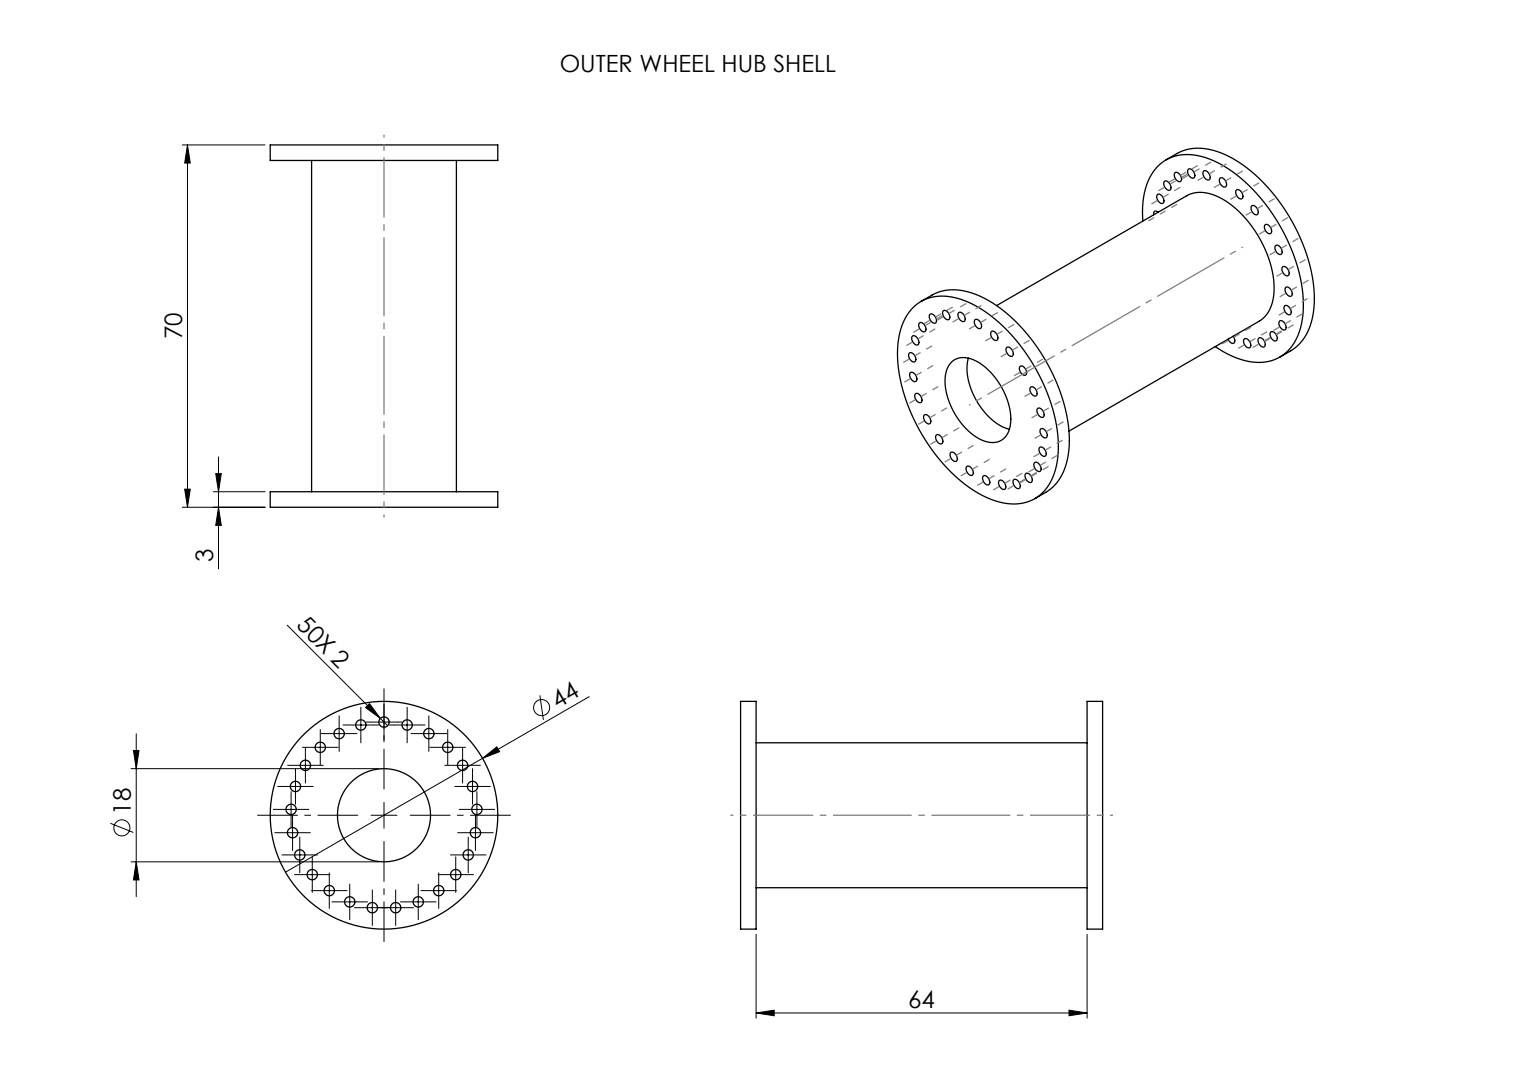
ISO-10303-21;
HEADER;
FILE_DESCRIPTION (('STEP AP214'),
    '1' );
FILE_NAME ('Outer Wheel Hub Shell.step',
    '2026-10-08T05:56:58',
    ( '' ),
    ( '' ),
    'SwSTEP 2.0',
    'SolidWorks 2026',
    '' );
FILE_SCHEMA (( 'AUTOMOTIVE_DESIGN' ));
ENDSEC;

DATA;
#6=ORIENTED_EDGE ( 'NONE', *, *, #9270, .F. ) ;
#16=VECTOR ( 'NONE', #6986, 1000.000000000000000 ) ;
#21=CARTESIAN_POINT ( 'NONE',  ( -14.19790265903626647, 9.644882309621941374, 35.00000000000000000 ) ) ;
#22=VERTEX_POINT ( 'NONE', #14244 ) ;
#27=DIRECTION ( 'NONE',  ( 0.000000000000000000, 0.000000000000000000, 1.000000000000000000 ) ) ;
#28=CARTESIAN_POINT ( 'NONE',  ( -10.58013454126452224, -14.56230589874905235, 32.00000000000000000 ) ) ;
#30=ORIENTED_EDGE ( 'NONE', *, *, #18526, .T. ) ;
#35=ADVANCED_FACE ( 'NONE', ( #2227 ), #2033, .F. ) ;
#38=CARTESIAN_POINT ( 'NONE',  ( 15.28688694438835505, -7.664027248171309203, -32.00000000000000000 ) ) ;
#40=ORIENTED_EDGE ( 'NONE', *, *, #11273, .T. ) ;
#42=ADVANCED_FACE ( 'NONE', ( #15944 ), #11240, .F. ) ;
#44=ORIENTED_EDGE ( 'NONE', *, *, #4692, .F. ) ;
#45=DIRECTION ( 'NONE',  ( 0.000000000000000000, 0.000000000000000000, -1.000000000000000000 ) ) ;
#52=CIRCLE ( 'NONE', #15065, 1.000000000000004441 ) ;
#61=AXIS2_PLACEMENT_3D ( 'NONE', #11825, #841, #14548 ) ;
#65=AXIS2_PLACEMENT_3D ( 'NONE', #16794, #19682, #3071 ) ;
#66=DIRECTION ( 'NONE',  ( -1.000000000000000000, 0.000000000000000000, 0.000000000000000000 ) ) ;
#68=DIRECTION ( 'NONE',  ( 1.000000000000000000, 0.000000000000000000, 0.000000000000000000 ) ) ;
#74=EDGE_CURVE ( 'NONE', #13547, #344, #8025, .T. ) ;
#78=FACE_BOUND ( 'NONE', #16173, .T. ) ;
#84=EDGE_CURVE ( 'NONE', #8438, #18497, #5035, .T. ) ;
#92=AXIS2_PLACEMENT_3D ( 'NONE', #12278, #16979, #66 ) ;
#99=CYLINDRICAL_SURFACE ( 'NONE', #7805, 22.00000000000000355 ) ;
#102=ORIENTED_EDGE ( 'NONE', *, *, #9565, .F. ) ;
#108=CARTESIAN_POINT ( 'NONE',  ( 0.000000000000000000, 0.000000000000000000, 35.00000000000000000 ) ) ;
#110=CARTESIAN_POINT ( 'NONE',  ( 17.11901729331276556, 5.562305898749055011, -32.00000000000000000 ) ) ;
#111=EDGE_CURVE ( 'NONE', #18625, #19430, #2327, .T. ) ;
#124=EDGE_CURVE ( 'NONE', #6609, #1230, #1374, .T. ) ;
#127=EDGE_CURVE ( 'NONE', #15888, #11336, #18737, .T. ) ;
#128=DIRECTION ( 'NONE',  ( 0.000000000000000000, 0.000000000000000000, 1.000000000000000000 ) ) ;
#129=ORIENTED_EDGE ( 'NONE', *, *, #9030, .F. ) ;
#130=DIRECTION ( 'NONE',  ( 1.000000000000000000, 0.000000000000000000, 0.000000000000000000 ) ) ;
#133=DIRECTION ( 'NONE',  ( 1.000000000000000000, 0.000000000000000000, 0.000000000000000000 ) ) ;
#143=DIRECTION ( 'NONE',  ( -0.000000000000000000, -0.000000000000000000, 1.000000000000000000 ) ) ;
#151=ORIENTED_EDGE ( 'NONE', *, *, #9100, .T. ) ;
#152=SHAPE_DEFINITION_REPRESENTATION ( #11949, #13463 ) ;
#155=VERTEX_POINT ( 'NONE', #3633 ) ;
#160=AXIS2_PLACEMENT_3D ( 'NONE', #12502, #14297, #392 ) ;
#165=VECTOR ( 'NONE', #11258, 1000.000000000000000 ) ;
#177=EDGE_LOOP ( 'NONE', ( #14869, #8807, #10159, #6951 ) ) ;
#183=DIRECTION ( 'NONE',  ( 0.000000000000000000, 0.000000000000000000, 1.000000000000000000 ) ) ;
#188=ORIENTED_EDGE ( 'NONE', *, *, #15203, .F. ) ;
#195=CARTESIAN_POINT ( 'NONE',  ( 12.86923836996420967, -11.47363181547641453, 32.00000000000000000 ) ) ;
#205=DIRECTION ( 'NONE',  ( 1.000000000000000000, 0.000000000000000000, 0.000000000000000000 ) ) ;
#209=ADVANCED_FACE ( 'NONE', ( #15358 ), #16764, .F. ) ;
#218=ORIENTED_EDGE ( 'NONE', *, *, #8182, .T. ) ;
#219=CIRCLE ( 'NONE', #8203, 1.000000000000000888 ) ;
#226=VERTEX_POINT ( 'NONE', #15455 ) ;
#228=EDGE_LOOP ( 'NONE', ( #8346, #6074 ) ) ;
#236=DIRECTION ( 'NONE',  ( 1.000000000000000000, 0.000000000000000000, 0.000000000000000000 ) ) ;
#245=ORIENTED_EDGE ( 'NONE', *, *, #12939, .T. ) ;
#257=VERTEX_POINT ( 'NONE', #7635 ) ;
#258=DIRECTION ( 'NONE',  ( 0.000000000000000000, 0.000000000000000000, 1.000000000000000000 ) ) ;
#261=ORIENTED_EDGE ( 'NONE', *, *, #7786, .T. ) ;
#264=FACE_BOUND ( 'NONE', #19064, .T. ) ;
#271=VERTEX_POINT ( 'NONE', #7531 ) ;
#273=AXIS2_PLACEMENT_3D ( 'NONE', #16273, #13173, #8869 ) ;
#277=DIRECTION ( 'NONE',  ( 1.000000000000000000, 0.000000000000000000, 0.000000000000000000 ) ) ;
#286=EDGE_CURVE ( 'NONE', #5172, #4659, #9375, .T. ) ;
#288=AXIS2_PLACEMENT_3D ( 'NONE', #4753, #9067, #13763 ) ;
#293=DIRECTION ( 'NONE',  ( 1.000000000000000000, 0.000000000000000000, 0.000000000000000000 ) ) ;
#295=DIRECTION ( 'NONE',  ( -1.000000000000000000, 0.000000000000000000, 0.000000000000000000 ) ) ;
#297=SURFACE_STYLE_FILL_AREA ( #4139 ) ;
#300=CARTESIAN_POINT ( 'NONE',  ( -18.11901729331277267, 5.562305898749051458, 35.00000000000000000 ) ) ;
#304=LINE ( 'NONE', #1515, #19226 ) ;
#305=CIRCLE ( 'NONE', #5078, 0.9999999999999974465 ) ;
#310=CYLINDRICAL_SURFACE ( 'NONE', #17454, 1.000000000000000888 ) ;
#319=CARTESIAN_POINT ( 'NONE',  ( 5.510910596163084625E-16, 18.00000000000000355, 32.00000000000000000 ) ) ;
#321=ORIENTED_EDGE ( 'NONE', *, *, #19741, .T. ) ;
#325=CYLINDRICAL_SURFACE ( 'NONE', #16943, 1.000000000000000888 ) ;
#330=ORIENTED_EDGE ( 'NONE', *, *, #12182, .F. ) ;
#341=CARTESIAN_POINT ( 'NONE',  ( 5.510910596163084625E-16, 18.00000000000000355, -32.00000000000000000 ) ) ;
#342=EDGE_LOOP ( 'NONE', ( #5793, #6421, #6456, #12755 ) ) ;
#344=VERTEX_POINT ( 'NONE', #2135 ) ;
#350=AXIS2_PLACEMENT_3D ( 'NONE', #15262, #4448, #9055 ) ;
#355=ORIENTED_EDGE ( 'NONE', *, *, #12536, .T. ) ;
#357=CARTESIAN_POINT ( 'NONE',  ( 14.00000000000000178, 1.714505518806294835E-15, -32.00000000000000000 ) ) ;
#360=FACE_OUTER_BOUND ( 'NONE', #7817, .T. ) ;
#362=CARTESIAN_POINT ( 'NONE',  ( 18.68117051311639543, -3.372863662543048591, 35.00000000000000000 ) ) ;
#365=ADVANCED_FACE ( 'NONE', ( #12843 ), #6521, .F. ) ;
#372=AXIS2_PLACEMENT_3D ( 'NONE', #16435, #19135, #4224 ) ;
#383=LINE ( 'NONE', #6367, #16649 ) ;
#388=AXIS2_PLACEMENT_3D ( 'NONE', #15598, #18590, #11093 ) ;
#389=AXIS2_PLACEMENT_3D ( 'NONE', #8278, #3775, #11481 ) ;
#390=CARTESIAN_POINT ( 'NONE',  ( -6.626241948324210540, -16.73597674598852336, 32.00000000000000000 ) ) ;
#392=DIRECTION ( 'NONE',  ( 1.000000000000000000, 0.000000000000000000, 0.000000000000000000 ) ) ;
#402=DIRECTION ( 'NONE',  ( 0.000000000000000000, 0.000000000000000000, -1.000000000000000000 ) ) ;
#404=CYLINDRICAL_SURFACE ( 'NONE', #4852, 1.000000000000004441 ) ;
#412=CIRCLE ( 'NONE', #11553, 1.000000000000004441 ) ;
#417=ORIENTED_EDGE ( 'NONE', *, *, #7596, .F. ) ;
#421=FACE_OUTER_BOUND ( 'NONE', #11319, .T. ) ;
#424=CARTESIAN_POINT ( 'NONE',  ( -9.580134541264520465, -14.56230589874905235, -35.00000000000000000 ) ) ;
#425=AXIS2_PLACEMENT_3D ( 'NONE', #7432, #4154, #17966 ) ;
#430=CARTESIAN_POINT ( 'NONE',  ( 17.68117051311639898, -3.372863662543048591, -32.00000000000000000 ) ) ;
#435=ORIENTED_EDGE ( 'NONE', *, *, #17905, .F. ) ;
#440=EDGE_LOOP ( 'NONE', ( #15883, #17623 ) ) ;
#454=ORIENTED_EDGE ( 'NONE', *, *, #8309, .T. ) ;
#459=ORIENTED_EDGE ( 'NONE', *, *, #7878, .F. ) ;
#468=ORIENTED_EDGE ( 'NONE', *, *, #6736, .T. ) ;
#473=DIRECTION ( 'NONE',  ( 0.000000000000000000, 0.000000000000000000, -1.000000000000000000 ) ) ;
#474=ORIENTED_EDGE ( 'NONE', *, *, #11666, .T. ) ;
#477=AXIS2_PLACEMENT_3D ( 'NONE', #18214, #19704, #4602 ) ;
#478=ORIENTED_EDGE ( 'NONE', *, *, #16286, .F. ) ;
#482=VECTOR ( 'NONE', #13106, 1000.000000000000000 ) ;
#490=ADVANCED_FACE ( 'NONE', ( #16238 ), #3832, .F. ) ;
#497=ORIENTED_EDGE ( 'NONE', *, *, #6656, .F. ) ;
#498=CIRCLE ( 'NONE', #11670, 0.9999999999999974465 ) ;
#499=DIRECTION ( 'NONE',  ( 1.000000000000000000, 0.000000000000000000, 0.000000000000000000 ) ) ;
#505=DIRECTION ( 'NONE',  ( 1.000000000000000000, 0.000000000000000000, 0.000000000000000000 ) ) ;
#511=CARTESIAN_POINT ( 'NONE',  ( 0.000000000000000000, 0.000000000000000000, -30.00000000000000355 ) ) ;
#512=ORIENTED_EDGE ( 'NONE', *, *, #15204, .T. ) ;
#518=FACE_OUTER_BOUND ( 'NONE', #1664, .T. ) ;
#521=CARTESIAN_POINT ( 'NONE',  ( -12.86923836996420611, -11.47363181547641275, 35.00000000000000000 ) ) ;
#524=CARTESIAN_POINT ( 'NONE',  ( -17.96448111170888851, 1.130229351527647585, 32.00000000000000000 ) ) ;
#526=DIRECTION ( 'NONE',  ( 0.000000000000000000, 0.000000000000000000, 1.000000000000000000 ) ) ;
#538=CARTESIAN_POINT ( 'NONE',  ( 12.32184790671639618, 13.12143529358541016, 32.00000000000000000 ) ) ;
#556=ORIENTED_EDGE ( 'NONE', *, *, #11604, .T. ) ;
#557=CARTESIAN_POINT ( 'NONE',  ( -12.00000000000000178, 0.000000000000000000, 35.00000000000000000 ) ) ;
#562=VERTEX_POINT ( 'NONE', #12229 ) ;
#563=DIRECTION ( 'NONE',  ( -0.000000000000000000, -0.000000000000000000, 1.000000000000000000 ) ) ;
#567=CIRCLE ( 'NONE', #11727, 14.00000000000000178 ) ;
#574=FACE_BOUND ( 'NONE', #7715, .T. ) ;
#584=DIRECTION ( 'NONE',  ( 0.000000000000000000, 0.000000000000000000, -1.000000000000000000 ) ) ;
#585=VECTOR ( 'NONE', #11111, 1000.000000000000000 ) ;
#586=ORIENTED_EDGE ( 'NONE', *, *, #6888, .T. ) ;
#587=CARTESIAN_POINT ( 'NONE',  ( -8.671566133830875600, 15.77352024078954429, -35.00000000000000000 ) ) ;
#597=CYLINDRICAL_SURFACE ( 'NONE', #3082, 1.000000000000004441 ) ;
#600=VERTEX_POINT ( 'NONE', #1222 ) ;
#601=CYLINDRICAL_SURFACE ( 'NONE', #13048, 1.000000000000000888 ) ;
#612=CARTESIAN_POINT ( 'NONE',  ( -12.32184790671639085, 13.12143529358541549, -32.00000000000000000 ) ) ;
#613=AXIS2_PLACEMENT_3D ( 'NONE', #10764, #563, #14261 ) ;
#620=CARTESIAN_POINT ( 'NONE',  ( -6.626241948324210540, -16.73597674598852336, -32.00000000000000000 ) ) ;
#625=ORIENTED_EDGE ( 'NONE', *, *, #10006, .T. ) ;
#636=FACE_BOUND ( 'NONE', #2747, .T. ) ;
#642=LINE ( 'NONE', #1837, #19205 ) ;
#649=EDGE_LOOP ( 'NONE', ( #15973, #2519, #13118, #2689 ) ) ;
#656=EDGE_LOOP ( 'NONE', ( #12086, #15329 ) ) ;
#662=EDGE_CURVE ( 'NONE', #16700, #600, #4069, .T. ) ;
#666=ORIENTED_EDGE ( 'NONE', *, *, #14685, .T. ) ;
#669=ADVANCED_FACE ( 'NONE', ( #3317 ), #12722, .F. ) ;
#672=ORIENTED_EDGE ( 'NONE', *, *, #13623, .F. ) ;
#674=LINE ( 'NONE', #2526, #7891 ) ;
#676=VERTEX_POINT ( 'NONE', #5011 ) ;
#705=ORIENTED_EDGE ( 'NONE', *, *, #2287, .T. ) ;
#711=ORIENTED_EDGE ( 'NONE', *, *, #7911, .F. ) ;
#716=AXIS2_PLACEMENT_3D ( 'NONE', #3976, #1170, #14686 ) ;
#718=CARTESIAN_POINT ( 'NONE',  ( 9.671566133830877376, 15.77352024078954784, -32.00000000000000000 ) ) ;
#722=FILL_AREA_STYLE_COLOUR ( '', #9371 ) ;
#726=DIRECTION ( 'NONE',  ( -1.000000000000000000, 0.000000000000000000, 0.000000000000000000 ) ) ;
#733=DIRECTION ( 'NONE',  ( 0.000000000000000000, 0.000000000000000000, -1.000000000000000000 ) ) ;
#735=DIRECTION ( 'NONE',  ( 1.000000000000000000, 0.000000000000000000, 0.000000000000000000 ) ) ;
#738=FACE_BOUND ( 'NONE', #4707, .T. ) ;
#742=CARTESIAN_POINT ( 'NONE',  ( -11.58013454126452579, -14.56230589874905235, -32.00000000000000000 ) ) ;
#743=DIRECTION ( 'NONE',  ( 0.000000000000000000, 0.000000000000000000, -1.000000000000000000 ) ) ;
#744=EDGE_CURVE ( 'NONE', #18193, #12621, #16104, .T. ) ;
#749=DIRECTION ( 'NONE',  ( 1.000000000000000000, 0.000000000000000000, 0.000000000000000000 ) ) ;
#753=AXIS2_PLACEMENT_3D ( 'NONE', #9858, #9653, #15648 ) ;
#764=ORIENTED_EDGE ( 'NONE', *, *, #5632, .T. ) ;
#770=CARTESIAN_POINT ( 'NONE',  ( -18.96448111170889206, 1.130229351527647585, -35.00000000000000000 ) ) ;
#771=DIRECTION ( 'NONE',  ( 0.000000000000000000, 0.000000000000000000, 1.000000000000000000 ) ) ;
#792=DIRECTION ( 'NONE',  ( 0.000000000000000000, 0.000000000000000000, 1.000000000000000000 ) ) ;
#797=CARTESIAN_POINT ( 'NONE',  ( -15.19790265903627180, 9.644882309621941374, 35.00000000000000000 ) ) ;
#799=CARTESIAN_POINT ( 'NONE',  ( -9.000000000000001776, 0.000000000000000000, -30.00000000000000355 ) ) ;
#823=DIRECTION ( 'NONE',  ( 1.000000000000000000, 0.000000000000000000, 0.000000000000000000 ) ) ;
#829=CARTESIAN_POINT ( 'NONE',  ( -16.28688694438836038, -7.664027248171298545, -32.00000000000000000 ) ) ;
#833=DIRECTION ( 'NONE',  ( -0.000000000000000000, -0.000000000000000000, 1.000000000000000000 ) ) ;
#834=AXIS2_PLACEMENT_3D ( 'NONE', #19075, #17680, #9988 ) ;
#837=FACE_BOUND ( 'NONE', #6605, .T. ) ;
#841=DIRECTION ( 'NONE',  ( -0.000000000000000000, -0.000000000000000000, 1.000000000000000000 ) ) ;
#846=FACE_BOUND ( 'NONE', #14940, .T. ) ;
#855=DIRECTION ( 'NONE',  ( 1.000000000000000000, 0.000000000000000000, 0.000000000000000000 ) ) ;
#857=ORIENTED_EDGE ( 'NONE', *, *, #17755, .F. ) ;
#865=DIRECTION ( 'NONE',  ( 0.000000000000000000, 0.000000000000000000, -1.000000000000000000 ) ) ;
#888=CARTESIAN_POINT ( 'NONE',  ( 3.476417968967386418, 17.43449690031536292, 32.00000000000000000 ) ) ;
#894=AXIS2_PLACEMENT_3D ( 'NONE', #13584, #13287, #16392 ) ;
#907=AXIS2_PLACEMENT_3D ( 'NONE', #1856, #14055, #13963 ) ;
#912=DIRECTION ( 'NONE',  ( 1.000000000000000000, 0.000000000000000000, 0.000000000000000000 ) ) ;
#916=ORIENTED_EDGE ( 'NONE', *, *, #8748, .F. ) ;
#928=DIRECTION ( 'NONE',  ( -1.000000000000000000, 0.000000000000000000, 0.000000000000000000 ) ) ;
#929=ORIENTED_EDGE ( 'NONE', *, *, #16286, .T. ) ;
#932=DIRECTION ( 'NONE',  ( 1.000000000000000000, 0.000000000000000000, 0.000000000000000000 ) ) ;
#933=AXIS2_PLACEMENT_3D ( 'NONE', #6535, #2148, #5051 ) ;
#936=DIRECTION ( 'NONE',  ( 1.000000000000000000, 0.000000000000000000, 0.000000000000000000 ) ) ;
#937=CARTESIAN_POINT ( 'NONE',  ( 0.000000000000000000, 0.000000000000000000, 35.00000000000000000 ) ) ;
#943=DIRECTION ( 'NONE',  ( 0.000000000000000000, 0.000000000000000000, -1.000000000000000000 ) ) ;
#945=LINE ( 'NONE', #13146, #9312 ) ;
#949=DIRECTION ( 'NONE',  ( -0.000000000000000000, -0.000000000000000000, 1.000000000000000000 ) ) ;
#953=ORIENTED_EDGE ( 'NONE', *, *, #8960, .T. ) ;
#961=ORIENTED_EDGE ( 'NONE', *, *, #11015, .T. ) ;
#962=CARTESIAN_POINT ( 'NONE',  ( 18.68117051311639543, -3.372863662543048591, 32.00000000000000000 ) ) ;
#963=CIRCLE ( 'NONE', #1919, 1.000000000000000888 ) ;
#967=DIRECTION ( 'NONE',  ( -1.000000000000000000, 0.000000000000000000, 0.000000000000000000 ) ) ;
#968=ORIENTED_EDGE ( 'NONE', *, *, #18592, .F. ) ;
#970=LINE ( 'NONE', #17684, #14905 ) ;
#971=ORIENTED_EDGE ( 'NONE', *, *, #4682, .F. ) ;
#982=DIRECTION ( 'NONE',  ( 0.000000000000000000, 0.000000000000000000, 1.000000000000000000 ) ) ;
#983=ORIENTED_EDGE ( 'NONE', *, *, #2761, .F. ) ;
#984=DIRECTION ( 'NONE',  ( 1.000000000000000000, 0.000000000000000000, 0.000000000000000000 ) ) ;
#996=ORIENTED_EDGE ( 'NONE', *, *, #13001, .F. ) ;
#1006=ORIENTED_EDGE ( 'NONE', *, *, #16529, .F. ) ;
#1009=CARTESIAN_POINT ( 'NONE',  ( 1.255998204157470211, -17.85806462366060288, 32.00000000000000000 ) ) ;
#1014=FACE_BOUND ( 'NONE', #7800, .T. ) ;
#1017=ORIENTED_EDGE ( 'NONE', *, *, #19676, .T. ) ;
#1019=EDGE_CURVE ( 'NONE', #15780, #17520, #11302, .T. ) ;
#1024=ORIENTED_EDGE ( 'NONE', *, *, #3666, .F. ) ;
#1027=ADVANCED_FACE ( 'NONE', ( #17294 ), #1697, .F. ) ;
#1028=FACE_OUTER_BOUND ( 'NONE', #19195, .T. ) ;
#1036=VECTOR ( 'NONE', #16677, 1000.000000000000000 ) ;
#1041=VERTEX_POINT ( 'NONE', #3291 ) ;
#1042=DIRECTION ( 'NONE',  ( -0.000000000000000000, -0.000000000000000000, 1.000000000000000000 ) ) ;
#1045=EDGE_LOOP ( 'NONE', ( #18049, #2720, #5129, #19018 ) ) ;
#1058=EDGE_LOOP ( 'NONE', ( #17820, #7756, #19150, #14489 ) ) ;
#1064=DIRECTION ( 'NONE',  ( 0.000000000000000000, 0.000000000000000000, 1.000000000000000000 ) ) ;
#1065=MECHANICAL_DESIGN_GEOMETRIC_PRESENTATION_REPRESENTATION('',(#9705),#3287);
#1066=EDGE_CURVE ( 'NONE', #1381, #19705, #15773, .T. ) ;
#1071=DIRECTION ( 'NONE',  ( 0.000000000000000000, 0.000000000000000000, -1.000000000000000000 ) ) ;
#1074=CARTESIAN_POINT ( 'NONE',  ( 15.19790265903627358, 9.644882309621939598, 32.00000000000000000 ) ) ;
#1076=CARTESIAN_POINT ( 'NONE',  ( -14.86923836996421144, -11.47363181547641275, 35.00000000000000000 ) ) ;
#1079=CARTESIAN_POINT ( 'NONE',  ( -13.86923836996420967, -11.47363181547641275, 32.00000000000000000 ) ) ;
#1084=CARTESIAN_POINT ( 'NONE',  ( 17.68117051311639898, -3.372863662543048591, 35.00000000000000000 ) ) ;
#1095=ORIENTED_EDGE ( 'NONE', *, *, #14831, .F. ) ;
#1098=DIRECTION ( 'NONE',  ( 1.000000000000000000, 0.000000000000000000, 0.000000000000000000 ) ) ;
#1101=CIRCLE ( 'NONE', #14213, 12.00000000000000178 ) ;
#1108=AXIS2_PLACEMENT_3D ( 'NONE', #4038, #19235, #5530 ) ;
#1115=CIRCLE ( 'NONE', #11348, 1.000000000000004441 ) ;
#1116=CARTESIAN_POINT ( 'NONE',  ( 17.96448111170888851, 1.130229351527639148, 35.00000000000000000 ) ) ;
#1117=DIRECTION ( 'NONE',  ( -1.000000000000000000, 0.000000000000000000, 0.000000000000000000 ) ) ;
#1124=ORIENTED_EDGE ( 'NONE', *, *, #12744, .T. ) ;
#1125=EDGE_CURVE ( 'NONE', #3988, #14268, #7776, .T. ) ;
#1129=VERTEX_POINT ( 'NONE', #6182 ) ;
#1143=EDGE_CURVE ( 'NONE', #7513, #15780, #9300, .T. ) ;
#1149=EDGE_CURVE ( 'NONE', #19757, #19457, #12600, .T. ) ;
#1151=DIRECTION ( 'NONE',  ( 1.000000000000000000, 0.000000000000000000, 0.000000000000000000 ) ) ;
#1152=AXIS2_PLACEMENT_3D ( 'NONE', #13149, #10064, #16167 ) ;
#1154=CARTESIAN_POINT ( 'NONE',  ( 17.11901729331276556, 5.562305898749055011, -35.00000000000000000 ) ) ;
#1161=ORIENTED_EDGE ( 'NONE', *, *, #6150, .T. ) ;
#1163=DIRECTION ( 'NONE',  ( 1.000000000000000000, 0.000000000000000000, 0.000000000000000000 ) ) ;
#1167=ORIENTED_EDGE ( 'NONE', *, *, #17905, .T. ) ;
#1170=DIRECTION ( 'NONE',  ( -0.000000000000000000, -0.000000000000000000, 1.000000000000000000 ) ) ;
#1172=ORIENTED_EDGE ( 'NONE', *, *, #662, .F. ) ;
#1175=CIRCLE ( 'NONE', #9821, 1.000000000000004441 ) ;
#1176=DIRECTION ( 'NONE',  ( 0.000000000000000000, 0.000000000000000000, -1.000000000000000000 ) ) ;
#1182=ORIENTED_EDGE ( 'NONE', *, *, #6055, .F. ) ;
#1183=FACE_OUTER_BOUND ( 'NONE', #8230, .T. ) ;
#1192=AXIS2_PLACEMENT_3D ( 'NONE', #12017, #18122, #12117 ) ;
#1194=DIRECTION ( 'NONE',  ( 1.000000000000000000, 0.000000000000000000, 0.000000000000000000 ) ) ;
#1202=DIRECTION ( 'NONE',  ( 1.000000000000000000, 0.000000000000000000, 0.000000000000000000 ) ) ;
#1203=CARTESIAN_POINT ( 'NONE',  ( -9.580134541264520465, -14.56230589874905235, -32.00000000000000000 ) ) ;
#1207=VERTEX_POINT ( 'NONE', #9905 ) ;
#1213=CYLINDRICAL_SURFACE ( 'NONE', #12720, 0.9999999999999974465 ) ;
#1216=DIRECTION ( 'NONE',  ( 1.000000000000000000, 0.000000000000000000, 0.000000000000000000 ) ) ;
#1220=CIRCLE ( 'NONE', #15590, 1.000000000000000000 ) ;
#1222=CARTESIAN_POINT ( 'NONE',  ( 1.000000000000003331, 18.00000000000000355, -32.00000000000000000 ) ) ;
#1225=CARTESIAN_POINT ( 'NONE',  ( -5.476417968967388639, 17.43449690031536292, 35.00000000000000000 ) ) ;
#1230=VERTEX_POINT ( 'NONE', #16099 ) ;
#1245=ORIENTED_EDGE ( 'NONE', *, *, #9812, .F. ) ;
#1249=CARTESIAN_POINT ( 'NONE',  ( -16.11901729331276911, 5.562305898749051458, -32.00000000000000000 ) ) ;
#1254=ORIENTED_EDGE ( 'NONE', *, *, #6270, .F. ) ;
#1260=EDGE_LOOP ( 'NONE', ( #13516, #17218, #40, #9749 ) ) ;
#1261=CYLINDRICAL_SURFACE ( 'NONE', #273, 1.000000000000004441 ) ;
#1268=DIRECTION ( 'NONE',  ( 1.000000000000000000, 0.000000000000000000, 0.000000000000000000 ) ) ;
#1273=CARTESIAN_POINT ( 'NONE',  ( 17.96448111170888851, 1.130229351527639148, 32.00000000000000000 ) ) ;
#1276=ADVANCED_FACE ( 'NONE', ( #9805 ), #15898, .F. ) ;
#1280=AXIS2_PLACEMENT_3D ( 'NONE', #15135, #2719, #4426 ) ;
#1285=FACE_BOUND ( 'NONE', #3109, .T. ) ;
#1286=DIRECTION ( 'NONE',  ( -0.000000000000000000, -0.000000000000000000, 1.000000000000000000 ) ) ;
#1289=ORIENTED_EDGE ( 'NONE', *, *, #15396, .F. ) ;
#1290=DIRECTION ( 'NONE',  ( 1.000000000000000000, 0.000000000000000000, 0.000000000000000000 ) ) ;
#1294=MECHANICAL_DESIGN_GEOMETRIC_PRESENTATION_REPRESENTATION('',(#18875),#16321);
#1307=VECTOR ( 'NONE', #11955, 1000.000000000000000 ) ;
#1310=DIRECTION ( 'NONE',  ( 1.000000000000000000, 0.000000000000000000, 0.000000000000000000 ) ) ;
#1326=ORIENTED_EDGE ( 'NONE', *, *, #18116, .T. ) ;
#1329=CARTESIAN_POINT ( 'NONE',  ( 9.580134541264516912, -14.56230589874905412, 32.00000000000000000 ) ) ;
#1332=DIRECTION ( 'NONE',  ( 1.000000000000000000, 0.000000000000000000, 0.000000000000000000 ) ) ;
#1348=DIRECTION ( 'NONE',  ( 1.000000000000000000, 0.000000000000000000, 0.000000000000000000 ) ) ;
#1355=DIRECTION ( 'NONE',  ( 0.000000000000000000, 0.000000000000000000, 1.000000000000000000 ) ) ;
#1356=ORIENTED_EDGE ( 'NONE', *, *, #6888, .F. ) ;
#1374=CIRCLE ( 'NONE', #3610, 1.000000000000000888 ) ;
#1381=VERTEX_POINT ( 'NONE', #7657 ) ;
#1383=CARTESIAN_POINT ( 'NONE',  ( 17.11901729331276556, 5.562305898749055011, -32.00000000000000000 ) ) ;
#1386=FACE_BOUND ( 'NONE', #8709, .T. ) ;
#1401=CARTESIAN_POINT ( 'NONE',  ( 17.28688694438834972, -7.664027248171309203, -32.00000000000000000 ) ) ;
#1405=ORIENTED_EDGE ( 'NONE', *, *, #10886, .T. ) ;
#1409=ORIENTED_EDGE ( 'NONE', *, *, #16598, .F. ) ;
#1433=CARTESIAN_POINT ( 'NONE',  ( -17.28688694438836393, -7.664027248171298545, 32.00000000000000000 ) ) ;
#1436=CARTESIAN_POINT ( 'NONE',  ( 16.68117051311640253, -3.372863662543048591, -32.00000000000000000 ) ) ;
#1440=EDGE_LOOP ( 'NONE', ( #2226, #11290, #7945, #5008 ) ) ;
#1441=DIRECTION ( 'NONE',  ( 1.000000000000000000, 0.000000000000000000, 0.000000000000000000 ) ) ;
#1445=EDGE_LOOP ( 'NONE', ( #3057, #18115, #929, #13564 ) ) ;
#1453=CARTESIAN_POINT ( 'NONE',  ( -7.671566133830872047, 15.77352024078954429, -32.00000000000000000 ) ) ;
#1459=DIRECTION ( 'NONE',  ( -0.000000000000000000, -0.000000000000000000, 1.000000000000000000 ) ) ;
#1466=DIRECTION ( 'NONE',  ( 0.000000000000000000, 0.000000000000000000, 1.000000000000000000 ) ) ;
#1470=DIRECTION ( 'NONE',  ( 1.000000000000000000, 0.000000000000000000, 0.000000000000000000 ) ) ;
#1479=FACE_OUTER_BOUND ( 'NONE', #9021, .T. ) ;
#1481=EDGE_CURVE ( 'NONE', #16968, #11811, #3329, .T. ) ;
#1482=CARTESIAN_POINT ( 'NONE',  ( 16.68117051311640253, -3.372863662543048591, -35.00000000000000000 ) ) ;
#1484=CARTESIAN_POINT ( 'NONE',  ( -16.11901729331276911, 5.562305898749051458, -32.00000000000000000 ) ) ;
#1495=VECTOR ( 'NONE', #5397, 1000.000000000000000 ) ;
#1500=EDGE_CURVE ( 'NONE', #17152, #9970, #8733, .T. ) ;
#1506=ORIENTED_EDGE ( 'NONE', *, *, #7570, .F. ) ;
#1509=DIRECTION ( 'NONE',  ( 0.000000000000000000, 0.000000000000000000, 1.000000000000000000 ) ) ;
#1511=DIRECTION ( 'NONE',  ( -1.000000000000000000, 0.000000000000000000, 0.000000000000000000 ) ) ;
#1515=CARTESIAN_POINT ( 'NONE',  ( 13.32184790671640151, 13.12143529358541016, 32.00000000000000000 ) ) ;
#1540=VERTEX_POINT ( 'NONE', #11540 ) ;
#1541=LINE ( 'NONE', #8480, #8395 ) ;
#1543=ORIENTED_EDGE ( 'NONE', *, *, #18666, .T. ) ;
#1544=ADVANCED_FACE ( 'NONE', ( #8450, #2523, #8633, #17836, #13425, #8542, #11832, #10345, #17940, #6924, #14553, #4229, #7304, #19523, #5815, #13045, #846, #16049, #14741, #11636, #2335, #17645, #4035, #3935, #10054, #1028, #16155 ), #14650, .T. ) ;
#1545=CARTESIAN_POINT ( 'NONE',  ( -16.28688694438836038, -7.664027248171298545, -35.00000000000000000 ) ) ;
#1561=VERTEX_POINT ( 'NONE', #4622 ) ;
#1564=ORIENTED_EDGE ( 'NONE', *, *, #9722, .T. ) ;
#1571=CIRCLE ( 'NONE', #15323, 1.000000000000002665 ) ;
#1579=FACE_BOUND ( 'NONE', #13672, .T. ) ;
#1594=EDGE_CURVE ( 'NONE', #15562, #8927, #9328, .T. ) ;
#1598=CARTESIAN_POINT ( 'NONE',  ( 9.000000000000001776, 1.102182119232617911E-15, -35.00000000000000000 ) ) ;
#1604=CARTESIAN_POINT ( 'NONE',  ( -12.32184790671639085, 13.12143529358541549, 35.00000000000000000 ) ) ;
#1622=ORIENTED_EDGE ( 'NONE', *, *, #5804, .T. ) ;
#1629=FACE_OUTER_BOUND ( 'NONE', #12937, .T. ) ;
#1632=EDGE_CURVE ( 'NONE', #7691, #8343, #10533, .T. ) ;
#1642=CARTESIAN_POINT ( 'NONE',  ( 2.255998204157473097, -17.85806462366060288, 32.00000000000000000 ) ) ;
#1643=ORIENTED_EDGE ( 'NONE', *, *, #12286, .T. ) ;
#1650=ORIENTED_EDGE ( 'NONE', *, *, #6270, .T. ) ;
#1651=PRODUCT_CONTEXT ( 'NONE', #13526, 'mechanical' ) ;
#1655=CIRCLE ( 'NONE', #5170, 1.000000000000002442 ) ;
#1657=EDGE_LOOP ( 'NONE', ( #2120, #15431 ) ) ;
#1664=EDGE_LOOP ( 'NONE', ( #2409, #12739, #5086, #102 ) ) ;
#1666=AXIS2_PLACEMENT_3D ( 'NONE', #16616, #18123, #1117 ) ;
#1668=CARTESIAN_POINT ( 'NONE',  ( -5.626241948324210540, -16.73597674598852336, -32.00000000000000000 ) ) ;
#1673=ORIENTED_EDGE ( 'NONE', *, *, #1481, .F. ) ;
#1678=ORIENTED_EDGE ( 'NONE', *, *, #6386, .F. ) ;
#1681=FACE_BOUND ( 'NONE', #14139, .T. ) ;
#1690=CARTESIAN_POINT ( 'NONE',  ( -14.86923836996421144, -11.47363181547641275, -32.00000000000000000 ) ) ;
#1697=CYLINDRICAL_SURFACE ( 'NONE', #17693, 1.000000000000005995 ) ;
#1703=CIRCLE ( 'NONE', #18636, 1.000000000000000888 ) ;
#1704=DIRECTION ( 'NONE',  ( 1.000000000000000000, 0.000000000000000000, 0.000000000000000000 ) ) ;
#1710=EDGE_CURVE ( 'NONE', #7772, #12395, #17396, .T. ) ;
#1720=VECTOR ( 'NONE', #1790, 1000.000000000000000 ) ;
#1724=DIRECTION ( 'NONE',  ( 0.000000000000000000, 0.000000000000000000, 1.000000000000000000 ) ) ;
#1728=EDGE_LOOP ( 'NONE', ( #2809, #13632, #15230, #15114 ) ) ;
#1731=DIRECTION ( 'NONE',  ( -0.000000000000000000, -0.000000000000000000, 1.000000000000000000 ) ) ;
#1732=DIRECTION ( 'NONE',  ( 0.000000000000000000, 0.000000000000000000, 1.000000000000000000 ) ) ;
#1737=ORIENTED_EDGE ( 'NONE', *, *, #18205, .F. ) ;
#1757=ORIENTED_EDGE ( 'NONE', *, *, #3055, .F. ) ;
#1761=ADVANCED_FACE ( 'NONE', ( #4820 ), #10928, .T. ) ;
#1764=DIRECTION ( 'NONE',  ( 1.000000000000000000, 0.000000000000000000, 0.000000000000000000 ) ) ;
#1765=AXIS2_PLACEMENT_3D ( 'NONE', #19492, #4393, #14903 ) ;
#1769=FACE_BOUND ( 'NONE', #11928, .T. ) ;
#1770=EDGE_LOOP ( 'NONE', ( #17052, #10177, #1780, #9726 ) ) ;
#1772=ORIENTED_EDGE ( 'NONE', *, *, #12734, .F. ) ;
#1774=CARTESIAN_POINT ( 'NONE',  ( 3.476417968967386418, 17.43449690031536292, -32.00000000000000000 ) ) ;
#1776=CARTESIAN_POINT ( 'NONE',  ( 12.32184790671639618, 13.12143529358541016, 35.00000000000000000 ) ) ;
#1777=AXIS2_PLACEMENT_3D ( 'NONE', #9171, #18934, #7926 ) ;
#1778=DIRECTION ( 'NONE',  ( 0.000000000000000000, 0.000000000000000000, 1.000000000000000000 ) ) ;
#1780=ORIENTED_EDGE ( 'NONE', *, *, #2004, .F. ) ;
#1783=ORIENTED_EDGE ( 'NONE', *, *, #13211, .F. ) ;
#1787=AXIS2_PLACEMENT_3D ( 'NONE', #3934, #10053, #936 ) ;
#1788=AXIS2_PLACEMENT_3D ( 'NONE', #612, #14017, #9523 ) ;
#1790=DIRECTION ( 'NONE',  ( 0.000000000000000000, 0.000000000000000000, 1.000000000000000000 ) ) ;
#1798=DIRECTION ( 'NONE',  ( 0.000000000000000000, 0.000000000000000000, 1.000000000000000000 ) ) ;
#1804=DIRECTION ( 'NONE',  ( 0.000000000000000000, 0.000000000000000000, 1.000000000000000000 ) ) ;
#1805=CIRCLE ( 'NONE', #9819, 1.000000000000002665 ) ;
#1812=DIRECTION ( 'NONE',  ( 0.000000000000000000, 0.000000000000000000, 1.000000000000000000 ) ) ;
#1813=EDGE_CURVE ( 'NONE', #6546, #2248, #12933, .T. ) ;
#1814=DIRECTION ( 'NONE',  ( -0.000000000000000000, -0.000000000000000000, 1.000000000000000000 ) ) ;
#1825=EDGE_LOOP ( 'NONE', ( #3083, #7794, #8665, #12430 ) ) ;
#1827=EDGE_CURVE ( 'NONE', #15645, #7691, #1101, .T. ) ;
#1832=DIRECTION ( 'NONE',  ( -1.000000000000000000, 0.000000000000000000, 0.000000000000000000 ) ) ;
#1833=AXIS2_PLACEMENT_3D ( 'NONE', #2667, #13476, #5869 ) ;
#1837=CARTESIAN_POINT ( 'NONE',  ( -9.000000000000001776, 0.000000000000000000, -30.00000000000000355 ) ) ;
#1840=EDGE_CURVE ( 'NONE', #11336, #8576, #19311, .T. ) ;
#1843=CARTESIAN_POINT ( 'NONE',  ( -18.11901729331277267, 5.562305898749051458, 32.00000000000000000 ) ) ;
#1845=DIRECTION ( 'NONE',  ( 0.000000000000000000, 0.000000000000000000, 1.000000000000000000 ) ) ;
#1847=CIRCLE ( 'NONE', #12704, 0.9999999999999974465 ) ;
#1848=ORIENTED_EDGE ( 'NONE', *, *, #17371, .F. ) ;
#1851=CIRCLE ( 'NONE', #14319, 1.000000000000004441 ) ;
#1855=EDGE_CURVE ( 'NONE', #10657, #10470, #19632, .T. ) ;
#1856=CARTESIAN_POINT ( 'NONE',  ( -10.58013454126452224, -14.56230589874905235, 35.00000000000000000 ) ) ;
#1861=ORIENTED_EDGE ( 'NONE', *, *, #5100, .F. ) ;
#1862=VECTOR ( 'NONE', #10499, 1000.000000000000000 ) ;
#1866=PLANE ( 'NONE',  #10369 ) ;
#1868=DIRECTION ( 'NONE',  ( 1.000000000000000000, 0.000000000000000000, 0.000000000000000000 ) ) ;
#1885=EDGE_CURVE ( 'NONE', #6940, #19582, #10071, .T. ) ;
#1890=ORIENTED_EDGE ( 'NONE', *, *, #9297, .F. ) ;
#1895=DIRECTION ( 'NONE',  ( 0.000000000000000000, 0.000000000000000000, 1.000000000000000000 ) ) ;
#1900=FACE_OUTER_BOUND ( 'NONE', #14171, .T. ) ;
#1919=AXIS2_PLACEMENT_3D ( 'NONE', #3428, #13935, #130 ) ;
#1920=EDGE_CURVE ( 'NONE', #16239, #12779, #9104, .T. ) ;
#1924=DIRECTION ( 'NONE',  ( 1.000000000000000000, 0.000000000000000000, 0.000000000000000000 ) ) ;
#1930=VECTOR ( 'NONE', #15016, 1000.000000000000000 ) ;
#1931=CARTESIAN_POINT ( 'NONE',  ( 17.96448111170888851, 1.130229351527639148, -32.00000000000000000 ) ) ;
#1932=ADVANCED_FACE ( 'NONE', ( #18310 ), #5989, .F. ) ;
#1935=ORIENTED_EDGE ( 'NONE', *, *, #10207, .F. ) ;
#1936=FACE_OUTER_BOUND ( 'NONE', #18621, .T. ) ;
#1939=CARTESIAN_POINT ( 'NONE',  ( -9.000000000000000000, 1.102182119232617714E-15, 29.00000000000000355 ) ) ;
#1950=ORIENTED_EDGE ( 'NONE', *, *, #11138, .T. ) ;
#1952=ADVANCED_FACE ( 'NONE', ( #10804 ), #99, .T. ) ;
#1955=EDGE_CURVE ( 'NONE', #6290, #5305, #9110, .T. ) ;
#1956=EDGE_CURVE ( 'NONE', #12131, #9602, #15813, .T. ) ;
#1958=AXIS2_PLACEMENT_3D ( 'NONE', #3030, #7628, #1441 ) ;
#1961=DIRECTION ( 'NONE',  ( -1.000000000000000000, 0.000000000000000000, 0.000000000000000000 ) ) ;
#1962=FACE_BOUND ( 'NONE', #8956, .T. ) ;
#1966=EDGE_LOOP ( 'NONE', ( #4725, #9031 ) ) ;
#1976=CARTESIAN_POINT ( 'NONE',  ( 0.000000000000000000, 0.000000000000000000, -30.00000000000000355 ) ) ;
#1977=VERTEX_POINT ( 'NONE', #1598 ) ;
#1979=ADVANCED_FACE ( 'NONE', ( #10512 ), #15111, .F. ) ;
#1983=DIRECTION ( 'NONE',  ( 1.000000000000000000, 0.000000000000000000, 0.000000000000000000 ) ) ;
#1987=CIRCLE ( 'NONE', #12226, 0.9999999999999974465 ) ;
#1990=CIRCLE ( 'NONE', #3591, 1.000000000000004441 ) ;
#1999=DIRECTION ( 'NONE',  ( 1.000000000000000000, 0.000000000000000000, 0.000000000000000000 ) ) ;
#2004=EDGE_CURVE ( 'NONE', #10647, #18235, #14855, .T. ) ;
#2012=DIRECTION ( 'NONE',  ( 1.000000000000000000, 0.000000000000000000, 0.000000000000000000 ) ) ;
#2023=VERTEX_POINT ( 'NONE', #1203 ) ;
#2024=DIRECTION ( 'NONE',  ( 0.000000000000000000, 0.000000000000000000, 1.000000000000000000 ) ) ;
#2025=DIRECTION ( 'NONE',  ( 0.000000000000000000, 0.000000000000000000, -1.000000000000000000 ) ) ;
#2033=CYLINDRICAL_SURFACE ( 'NONE', #12562, 1.000000000000000888 ) ;
#2034=DIRECTION ( 'NONE',  ( -0.000000000000000000, -0.000000000000000000, 1.000000000000000000 ) ) ;
#2036=ORIENTED_EDGE ( 'NONE', *, *, #17824, .T. ) ;
#2047=ORIENTED_EDGE ( 'NONE', *, *, #2731, .F. ) ;
#2064=VECTOR ( 'NONE', #19500, 1000.000000000000000 ) ;
#2073=ORIENTED_EDGE ( 'NONE', *, *, #10828, .T. ) ;
#2087=DIRECTION ( 'NONE',  ( 1.000000000000000000, 0.000000000000000000, 0.000000000000000000 ) ) ;
#2088=CIRCLE ( 'NONE', #4975, 1.000000000000002442 ) ;
#2091=ADVANCED_FACE ( 'NONE', ( #17202 ), #11099, .F. ) ;
#2092=DIRECTION ( 'NONE',  ( 0.000000000000000000, 0.000000000000000000, 1.000000000000000000 ) ) ;
#2097=EDGE_CURVE ( 'NONE', #4232, #5897, #15500, .T. ) ;
#2098=DIRECTION ( 'NONE',  ( 0.000000000000000000, 0.000000000000000000, -1.000000000000000000 ) ) ;
#2100=ORIENTED_EDGE ( 'NONE', *, *, #7221, .T. ) ;
#2103=CIRCLE ( 'NONE', #8817, 1.000000000000003553 ) ;
#2104=ORIENTED_EDGE ( 'NONE', *, *, #10242, .T. ) ;
#2106=CIRCLE ( 'NONE', #1777, 1.000000000000004441 ) ;
#2107=EDGE_CURVE ( 'NONE', #13012, #3997, #1115, .T. ) ;
#2113=ADVANCED_FACE ( 'NONE', ( #4992 ), #15699, .F. ) ;
#2116=DIRECTION ( 'NONE',  ( 0.000000000000000000, 0.000000000000000000, -1.000000000000000000 ) ) ;
#2120=ORIENTED_EDGE ( 'NONE', *, *, #16487, .T. ) ;
#2123=LINE ( 'NONE', #9640, #15256 ) ;
#2127=FACE_BOUND ( 'NONE', #19598, .T. ) ;
#2129=ORIENTED_EDGE ( 'NONE', *, *, #10476, .T. ) ;
#2131=AXIS2_PLACEMENT_3D ( 'NONE', #17009, #14003, #293 ) ;
#2135=CARTESIAN_POINT ( 'NONE',  ( -11.58013454126452579, -14.56230589874905235, -35.00000000000000000 ) ) ;
#2145=ORIENTED_EDGE ( 'NONE', *, *, #5100, .T. ) ;
#2148=DIRECTION ( 'NONE',  ( -0.000000000000000000, -0.000000000000000000, 1.000000000000000000 ) ) ;
#2149=CARTESIAN_POINT ( 'NONE',  ( -13.32184790671639618, 13.12143529358541549, -32.00000000000000000 ) ) ;
#2157=LINE ( 'NONE', #4763, #3488 ) ;
#2158=EDGE_CURVE ( 'NONE', #18514, #7536, #8780, .T. ) ;
#2163=DIRECTION ( 'NONE',  ( 1.000000000000000000, 0.000000000000000000, 0.000000000000000000 ) ) ;
#2165=ORIENTED_EDGE ( 'NONE', *, *, #14812, .T. ) ;
#2166=ORIENTED_EDGE ( 'NONE', *, *, #5206, .T. ) ;
#2173=ORIENTED_EDGE ( 'NONE', *, *, #13869, .T. ) ;
#2177=CARTESIAN_POINT ( 'NONE',  ( 16.68117051311640253, -3.372863662543048591, 32.00000000000000000 ) ) ;
#2178=DIRECTION ( 'NONE',  ( -1.000000000000000000, 0.000000000000000000, 0.000000000000000000 ) ) ;
#2180=DIRECTION ( 'NONE',  ( 1.000000000000000000, 0.000000000000000000, 0.000000000000000000 ) ) ;
#2181=CARTESIAN_POINT ( 'NONE',  ( -17.68117051311639898, -3.372863662543042818, 32.00000000000000000 ) ) ;
#2192=DIRECTION ( 'NONE',  ( 0.000000000000000000, 0.000000000000000000, 1.000000000000000000 ) ) ;
#2197=EDGE_CURVE ( 'NONE', #3237, #9521, #3579, .T. ) ;
#2199=CIRCLE ( 'NONE', #17217, 1.000000000000002665 ) ;
#2208=DIRECTION ( 'NONE',  ( 0.000000000000000000, 0.000000000000000000, -1.000000000000000000 ) ) ;
#2212=ORIENTED_EDGE ( 'NONE', *, *, #16965, .T. ) ;
#2223=DIRECTION ( 'NONE',  ( -0.000000000000000000, -0.000000000000000000, 1.000000000000000000 ) ) ;
#2226=ORIENTED_EDGE ( 'NONE', *, *, #5115, .F. ) ;
#2227=FACE_OUTER_BOUND ( 'NONE', #10980, .T. ) ;
#2231=EDGE_CURVE ( 'NONE', #11527, #16673, #17972, .T. ) ;
#2244=CARTESIAN_POINT ( 'NONE',  ( -4.476417968967385974, 17.43449690031536292, 32.00000000000000000 ) ) ;
#2246=DIRECTION ( 'NONE',  ( 0.000000000000000000, 0.000000000000000000, 1.000000000000000000 ) ) ;
#2248=VERTEX_POINT ( 'NONE', #11493 ) ;
#2252=ORIENTED_EDGE ( 'NONE', *, *, #1632, .F. ) ;
#2255=VECTOR ( 'NONE', #13804, 1000.000000000000000 ) ;
#2257=VERTEX_POINT ( 'NONE', #14602 ) ;
#2260=DIRECTION ( 'NONE',  ( 1.000000000000000000, 0.000000000000000000, 0.000000000000000000 ) ) ;
#2262=CIRCLE ( 'NONE', #9628, 0.9999999999999974465 ) ;
#2266=EDGE_CURVE ( 'NONE', #15965, #10636, #12899, .T. ) ;
#2267=EDGE_LOOP ( 'NONE', ( #2927, #12405 ) ) ;
#2269=CARTESIAN_POINT ( 'NONE',  ( 18.11901729331276911, 5.562305898749055011, 32.00000000000000000 ) ) ;
#2270=CARTESIAN_POINT ( 'NONE',  ( 17.96448111170888851, 1.130229351527639148, 35.00000000000000000 ) ) ;
#2272=LINE ( 'NONE', #10179, #11685 ) ;
#2283=CARTESIAN_POINT ( 'NONE',  ( -16.28688694438836038, -7.664027248171298545, 32.00000000000000000 ) ) ;
#2286=ORIENTED_EDGE ( 'NONE', *, *, #16716, .T. ) ;
#2287=EDGE_CURVE ( 'NONE', #18497, #9970, #14121, .T. ) ;
#2293=DIRECTION ( 'NONE',  ( 0.000000000000000000, 0.000000000000000000, 1.000000000000000000 ) ) ;
#2296=ORIENTED_EDGE ( 'NONE', *, *, #13115, .F. ) ;
#2302=AXIS2_PLACEMENT_3D ( 'NONE', #9106, #18305, #10602 ) ;
#2303=CIRCLE ( 'NONE', #9022, 1.000000000000002665 ) ;
#2307=DIRECTION ( 'NONE',  ( 0.000000000000000000, 0.000000000000000000, 1.000000000000000000 ) ) ;
#2315=ORIENTED_EDGE ( 'NONE', *, *, #3702, .F. ) ;
#2318=DIRECTION ( 'NONE',  ( 0.000000000000000000, 0.000000000000000000, 1.000000000000000000 ) ) ;
#2319=CIRCLE ( 'NONE', #15751, 1.000000000000000000 ) ;
#2327=CIRCLE ( 'NONE', #6156, 1.000000000000000888 ) ;
#2335=FACE_BOUND ( 'NONE', #13427, .T. ) ;
#2345=CARTESIAN_POINT ( 'NONE',  ( -15.28688694438835505, -7.664027248171298545, 32.00000000000000000 ) ) ;
#2348=DIRECTION ( 'NONE',  ( 1.000000000000000000, 0.000000000000000000, 0.000000000000000000 ) ) ;
#2356=EDGE_CURVE ( 'NONE', #15965, #6632, #7398, .T. ) ;
#2359=DIRECTION ( 'NONE',  ( 1.000000000000000000, 0.000000000000000000, 0.000000000000000000 ) ) ;
#2360=AXIS2_PLACEMENT_3D ( 'NONE', #14551, #9956, #15850 ) ;
#2364=ORIENTED_EDGE ( 'NONE', *, *, #11308, .T. ) ;
#2373=VECTOR ( 'NONE', #13954, 1000.000000000000000 ) ;
#2376=AXIS2_PLACEMENT_3D ( 'NONE', #16021, #4107, #11708 ) ;
#2377=FACE_OUTER_BOUND ( 'NONE', #7576, .T. ) ;
#2379=DIRECTION ( 'NONE',  ( -0.000000000000000000, -0.000000000000000000, 1.000000000000000000 ) ) ;
#2382=DIRECTION ( 'NONE',  ( 0.000000000000000000, 0.000000000000000000, 1.000000000000000000 ) ) ;
#2387=UNCERTAINTY_MEASURE_WITH_UNIT (LENGTH_MEASURE( 1.000000000000000082E-05 ), #7591, 'distance_accuracy_value', 'NONE');
#2395=ORIENTED_EDGE ( 'NONE', *, *, #2705, .T. ) ;
#2396=LINE ( 'NONE', #3899, #482 ) ;
#2399=CIRCLE ( 'NONE', #12641, 1.000000000000004441 ) ;
#2404=CARTESIAN_POINT ( 'NONE',  ( 0.000000000000000000, 0.000000000000000000, 35.00000000000000000 ) ) ;
#2409=ORIENTED_EDGE ( 'NONE', *, *, #13411, .T. ) ;
#2411=CARTESIAN_POINT ( 'NONE',  ( 0.000000000000000000, 0.000000000000000000, -32.00000000000000000 ) ) ;
#2412=DIRECTION ( 'NONE',  ( 1.000000000000000000, 0.000000000000000000, 0.000000000000000000 ) ) ;
#2414=CARTESIAN_POINT ( 'NONE',  ( -17.96448111170888851, 1.130229351527647585, -32.00000000000000000 ) ) ;
#2415=AXIS2_PLACEMENT_3D ( 'NONE', #16479, #13274, #15072 ) ;
#2419=VERTEX_POINT ( 'NONE', #5963 ) ;
#2420=CARTESIAN_POINT ( 'NONE',  ( 9.671566133830877376, 15.77352024078954784, -35.00000000000000000 ) ) ;
#2437=CARTESIAN_POINT ( 'NONE',  ( -16.19790265903627713, 9.644882309621941374, 35.00000000000000000 ) ) ;
#2438=ORIENTED_EDGE ( 'NONE', *, *, #6884, .T. ) ;
#2440=ADVANCED_FACE ( 'NONE', ( #1479 ), #15087, .F. ) ;
#2454=EDGE_LOOP ( 'NONE', ( #3809, #13101, #10322, #6636 ) ) ;
#2457=EDGE_CURVE ( 'NONE', #18074, #5711, #13490, .T. ) ;
#2458=CARTESIAN_POINT ( 'NONE',  ( -2.255998204157477538, -17.85806462366060288, 35.00000000000000000 ) ) ;
#2466=VECTOR ( 'NONE', #3155, 1000.000000000000000 ) ;
#2467=EDGE_CURVE ( 'NONE', #1561, #9666, #6442, .T. ) ;
#2487=ORIENTED_EDGE ( 'NONE', *, *, #6656, .T. ) ;
#2488=CARTESIAN_POINT ( 'NONE',  ( 0.000000000000000000, 0.000000000000000000, -30.00000000000000355 ) ) ;
#2489=ADVANCED_FACE ( 'NONE', ( #12287 ), #18089, .F. ) ;
#2501=DIRECTION ( 'NONE',  ( 0.000000000000000000, 0.000000000000000000, 1.000000000000000000 ) ) ;
#2505=ADVANCED_FACE ( 'NONE', ( #6649 ), #11985, .F. ) ;
#2507=CARTESIAN_POINT ( 'NONE',  ( 2.255998204157473097, -17.85806462366060288, 32.00000000000000000 ) ) ;
#2519=ORIENTED_EDGE ( 'NONE', *, *, #10327, .T. ) ;
#2523=FACE_BOUND ( 'NONE', #8452, .T. ) ;
#2526=CARTESIAN_POINT ( 'NONE',  ( 12.86923836996420967, -11.47363181547641453, -32.00000000000000000 ) ) ;
#2532=LINE ( 'NONE', #7024, #3158 ) ;
#2535=EDGE_LOOP ( 'NONE', ( #11441, #1161, #5372, #16742 ) ) ;
#2542=EDGE_LOOP ( 'NONE', ( #12122, #11121, #7342, #5440 ) ) ;
#2543=DIRECTION ( 'NONE',  ( -1.000000000000000000, 0.000000000000000000, 0.000000000000000000 ) ) ;
#2550=CIRCLE ( 'NONE', #12792, 0.9999999999999974465 ) ;
#2557=EDGE_CURVE ( 'NONE', #18644, #562, #3563, .T. ) ;
#2558=CYLINDRICAL_SURFACE ( 'NONE', #3258, 1.000000000000004441 ) ;
#2578=ORIENTED_EDGE ( 'NONE', *, *, #18821, .F. ) ;
#2591=AXIS2_PLACEMENT_3D ( 'NONE', #12649, #18642, #11146 ) ;
#2592=AXIS2_PLACEMENT_3D ( 'NONE', #19419, #5705, #19622 ) ;
#2593=DIRECTION ( 'NONE',  ( 0.000000000000000000, 0.000000000000000000, 1.000000000000000000 ) ) ;
#2595=CIRCLE ( 'NONE', #8359, 1.000000000000003109 ) ;
#2605=CYLINDRICAL_SURFACE ( 'NONE', #8560, 1.000000000000002665 ) ;
#2610=ORIENTED_EDGE ( 'NONE', *, *, #7522, .T. ) ;
#2612=AXIS2_PLACEMENT_3D ( 'NONE', #15614, #1804, #12217 ) ;
#2619=ORIENTED_EDGE ( 'NONE', *, *, #10872, .T. ) ;
#2621=EDGE_LOOP ( 'NONE', ( #968, #5215, #13361, #10275 ) ) ;
#2624=EDGE_LOOP ( 'NONE', ( #11380, #14427, #9352, #15291 ) ) ;
#2625=AXIS2_PLACEMENT_3D ( 'NONE', #8074, #17387, #3675 ) ;
#2630=CARTESIAN_POINT ( 'NONE',  ( 17.96448111170888851, 1.130229351527639148, -32.00000000000000000 ) ) ;
#2633=AXIS2_PLACEMENT_3D ( 'NONE', #12364, #9262, #12262 ) ;
#2635=DIRECTION ( 'NONE',  ( -0.000000000000000000, -0.000000000000000000, 1.000000000000000000 ) ) ;
#2637=ORIENTED_EDGE ( 'NONE', *, *, #3917, .F. ) ;
#2638=DIRECTION ( 'NONE',  ( 0.000000000000000000, 0.000000000000000000, 1.000000000000000000 ) ) ;
#2651=CYLINDRICAL_SURFACE ( 'NONE', #11136, 1.000000000000002665 ) ;
#2657=CARTESIAN_POINT ( 'NONE',  ( -15.19790265903627180, 9.644882309621941374, -32.00000000000000000 ) ) ;
#2662=EDGE_CURVE ( 'NONE', #4037, #9386, #15880, .T. ) ;
#2667=CARTESIAN_POINT ( 'NONE',  ( 13.86923836996420789, -11.47363181547641453, 32.00000000000000000 ) ) ;
#2668=DIRECTION ( 'NONE',  ( -0.000000000000000000, -0.000000000000000000, 1.000000000000000000 ) ) ;
#2669=EDGE_CURVE ( 'NONE', #2248, #6546, #11911, .T. ) ;
#2671=ORIENTED_EDGE ( 'NONE', *, *, #18158, .F. ) ;
#2676=CIRCLE ( 'NONE', #16434, 22.00000000000000355 ) ;
#2678=VERTEX_POINT ( 'NONE', #7038 ) ;
#2689=ORIENTED_EDGE ( 'NONE', *, *, #4751, .F. ) ;
#2690=AXIS2_PLACEMENT_3D ( 'NONE', #13346, #5544, #3953 ) ;
#2698=CYLINDRICAL_SURFACE ( 'NONE', #18844, 1.000000000000002665 ) ;
#2705=EDGE_CURVE ( 'NONE', #9559, #13272, #16076, .T. ) ;
#2712=CARTESIAN_POINT ( 'NONE',  ( 5.510910596163084625E-16, 18.00000000000000355, 32.00000000000000000 ) ) ;
#2719=DIRECTION ( 'NONE',  ( 0.000000000000000000, 0.000000000000000000, -1.000000000000000000 ) ) ;
#2720=ORIENTED_EDGE ( 'NONE', *, *, #12633, .T. ) ;
#2721=DIRECTION ( 'NONE',  ( 1.000000000000000000, 0.000000000000000000, 0.000000000000000000 ) ) ;
#2723=VERTEX_POINT ( 'NONE', #2947 ) ;
#2726=CARTESIAN_POINT ( 'NONE',  ( 7.671566133830872047, 15.77352024078954784, 32.00000000000000000 ) ) ;
#2727=CARTESIAN_POINT ( 'NONE',  ( -11.58013454126452579, -14.56230589874905235, -32.00000000000000000 ) ) ;
#2731=EDGE_CURVE ( 'NONE', #2257, #15969, #5945, .T. ) ;
#2732=CARTESIAN_POINT ( 'NONE',  ( 8.671566133830875600, 15.77352024078954784, -35.00000000000000000 ) ) ;
#2735=AXIS2_PLACEMENT_3D ( 'NONE', #3430, #6406, #1924 ) ;
#2738=DIRECTION ( 'NONE',  ( 1.000000000000000000, 0.000000000000000000, 0.000000000000000000 ) ) ;
#2743=CARTESIAN_POINT ( 'NONE',  ( 17.28688694438834972, -7.664027248171309203, -32.00000000000000000 ) ) ;
#2747=EDGE_LOOP ( 'NONE', ( #11610, #3472 ) ) ;
#2748=ORIENTED_EDGE ( 'NONE', *, *, #3055, .T. ) ;
#2749=CARTESIAN_POINT ( 'NONE',  ( 17.68117051311639898, -3.372863662543048591, 32.00000000000000000 ) ) ;
#2760=DIRECTION ( 'NONE',  ( -0.000000000000000000, -0.000000000000000000, 1.000000000000000000 ) ) ;
#2761=EDGE_CURVE ( 'NONE', #1129, #15138, #17026, .T. ) ;
#2771=CARTESIAN_POINT ( 'NONE',  ( -15.28688694438835505, -7.664027248171298545, 35.00000000000000000 ) ) ;
#2772=DIRECTION ( 'NONE',  ( -1.000000000000000000, 0.000000000000000000, 0.000000000000000000 ) ) ;
#2776=AXIS2_PLACEMENT_3D ( 'NONE', #16984, #3266, #15183 ) ;
#2777=CYLINDRICAL_SURFACE ( 'NONE', #6956, 14.00000000000000178 ) ;
#2780=DIRECTION ( 'NONE',  ( 0.000000000000000000, 0.000000000000000000, 1.000000000000000000 ) ) ;
#2783=VERTEX_POINT ( 'NONE', #6428 ) ;
#2785=EDGE_CURVE ( 'NONE', #8438, #17152, #19249, .T. ) ;
#2790=CIRCLE ( 'NONE', #13987, 1.000000000000002665 ) ;
#2795=ORIENTED_EDGE ( 'NONE', *, *, #5804, .F. ) ;
#2796=DIRECTION ( 'NONE',  ( 1.000000000000000000, 0.000000000000000000, 0.000000000000000000 ) ) ;
#2800=AXIS2_PLACEMENT_3D ( 'NONE', #8005, #1814, #2012 ) ;
#2809=ORIENTED_EDGE ( 'NONE', *, *, #15833, .F. ) ;
#2810=VECTOR ( 'NONE', #5879, 1000.000000000000000 ) ;
#2822=EDGE_LOOP ( 'NONE', ( #1772, #15376, #17903, #478 ) ) ;
#2837=EDGE_LOOP ( 'NONE', ( #2104, #1950 ) ) ;
#2845=CARTESIAN_POINT ( 'NONE',  ( 17.11901729331276556, 5.562305898749055011, 32.00000000000000000 ) ) ;
#2846=EDGE_LOOP ( 'NONE', ( #4452, #8328 ) ) ;
#2861=DIRECTION ( 'NONE',  ( 0.000000000000000000, 0.000000000000000000, -1.000000000000000000 ) ) ;
#2870=DIRECTION ( 'NONE',  ( 0.000000000000000000, 0.000000000000000000, -1.000000000000000000 ) ) ;
#2872=CARTESIAN_POINT ( 'NONE',  ( 15.19790265903627358, 9.644882309621939598, -32.00000000000000000 ) ) ;
#2878=ORIENTED_EDGE ( 'NONE', *, *, #16462, .T. ) ;
#2885=AXIS2_PLACEMENT_3D ( 'NONE', #9936, #2116, #726 ) ;
#2888=DIRECTION ( 'NONE',  ( 0.000000000000000000, 0.000000000000000000, 1.000000000000000000 ) ) ;
#2890=ORIENTED_EDGE ( 'NONE', *, *, #4836, .T. ) ;
#2897=EDGE_CURVE ( 'NONE', #13172, #11527, #18553, .T. ) ;
#2900=DIRECTION ( 'NONE',  ( 1.000000000000000000, 0.000000000000000000, 0.000000000000000000 ) ) ;
#2901=VERTEX_POINT ( 'NONE', #6628 ) ;
#2907=DIRECTION ( 'NONE',  ( 1.000000000000000000, 0.000000000000000000, 0.000000000000000000 ) ) ;
#2917=EDGE_LOOP ( 'NONE', ( #17953, #13648 ) ) ;
#2925=AXIS2_PLACEMENT_3D ( 'NONE', #7500, #7391, #1216 ) ;
#2927=ORIENTED_EDGE ( 'NONE', *, *, #18222, .F. ) ;
#2932=DIRECTION ( 'NONE',  ( 1.000000000000000000, 0.000000000000000000, 0.000000000000000000 ) ) ;
#2936=VECTOR ( 'NONE', #17518, 1000.000000000000000 ) ;
#2939=DIRECTION ( 'NONE',  ( -0.000000000000000000, -0.000000000000000000, 1.000000000000000000 ) ) ;
#2947=CARTESIAN_POINT ( 'NONE',  ( 13.32184790671640151, 13.12143529358541016, 32.00000000000000000 ) ) ;
#2949=ORIENTED_EDGE ( 'NONE', *, *, #1019, .F. ) ;
#2956=AXIS2_PLACEMENT_3D ( 'NONE', #1273, #5960, #7558 ) ;
#2959=CARTESIAN_POINT ( 'NONE',  ( -10.58013454126452224, -14.56230589874905235, 35.00000000000000000 ) ) ;
#2975=CARTESIAN_POINT ( 'NONE',  ( 14.00000000000000178, 1.714505518806294835E-15, 35.00000000000000000 ) ) ;
#2979=AXIS2_PLACEMENT_3D ( 'NONE', #7261, #5294, #11400 ) ;
#2980=DIRECTION ( 'NONE',  ( 0.000000000000000000, 0.000000000000000000, 1.000000000000000000 ) ) ;
#2987=VERTEX_POINT ( 'NONE', #7694 ) ;
#2995=DIRECTION ( 'NONE',  ( 1.000000000000000000, 0.000000000000000000, 0.000000000000000000 ) ) ;
#2997=DIRECTION ( 'NONE',  ( 1.000000000000000000, 0.000000000000000000, 0.000000000000000000 ) ) ;
#2998=AXIS2_PLACEMENT_3D ( 'NONE', #16100, #2379, #8493 ) ;
#3004=LINE ( 'NONE', #9119, #3451 ) ;
#3007=AXIS2_PLACEMENT_3D ( 'NONE', #18946, #15852, #749 ) ;
#3011=CIRCLE ( 'NONE', #14202, 1.000000000000000888 ) ;
#3012=EDGE_CURVE ( 'NONE', #10657, #6388, #9214, .T. ) ;
#3013=CARTESIAN_POINT ( 'NONE',  ( 17.68117051311639898, -3.372863662543048591, -35.00000000000000000 ) ) ;
#3024=FACE_OUTER_BOUND ( 'NONE', #11731, .T. ) ;
#3030=CARTESIAN_POINT ( 'NONE',  ( 15.19790265903627358, 9.644882309621939598, -35.00000000000000000 ) ) ;
#3035=DIRECTION ( 'NONE',  ( 0.000000000000000000, 0.000000000000000000, 1.000000000000000000 ) ) ;
#3037=VERTEX_POINT ( 'NONE', #10150 ) ;
#3043=SURFACE_STYLE_FILL_AREA ( #6799 ) ;
#3055=EDGE_CURVE ( 'NONE', #16700, #1129, #12317, .T. ) ;
#3056=CARTESIAN_POINT ( 'NONE',  ( 0.000000000000000000, 0.000000000000000000, -30.00000000000000355 ) ) ;
#3057=ORIENTED_EDGE ( 'NONE', *, *, #12490, .F. ) ;
#3059=DIRECTION ( 'NONE',  ( 0.000000000000000000, 0.000000000000000000, 1.000000000000000000 ) ) ;
#3063=CARTESIAN_POINT ( 'NONE',  ( -22.00000000000000355, 2.694222958124177204E-15, 35.00000000000000000 ) ) ;
#3071=DIRECTION ( 'NONE',  ( 1.000000000000000000, 0.000000000000000000, 0.000000000000000000 ) ) ;
#3075=FACE_BOUND ( 'NONE', #16640, .T. ) ;
#3077=DIRECTION ( 'NONE',  ( -0.000000000000000000, -0.000000000000000000, 1.000000000000000000 ) ) ;
#3082=AXIS2_PLACEMENT_3D ( 'NONE', #10000, #14196, #16102 ) ;
#3083=ORIENTED_EDGE ( 'NONE', *, *, #17542, .F. ) ;
#3088=CARTESIAN_POINT ( 'NONE',  ( 14.86923836996420434, -11.47363181547641453, 35.00000000000000000 ) ) ;
#3094=DIRECTION ( 'NONE',  ( -0.000000000000000000, -0.000000000000000000, 1.000000000000000000 ) ) ;
#3102=AXIS2_PLACEMENT_3D ( 'NONE', #13384, #19483, #2772 ) ;
#3104=ORIENTED_EDGE ( 'NONE', *, *, #4560, .T. ) ;
#3106=EDGE_CURVE ( 'NONE', #16740, #11695, #1703, .T. ) ;
#3109=EDGE_LOOP ( 'NONE', ( #14326, #16621 ) ) ;
#3117=VERTEX_POINT ( 'NONE', #3401 ) ;
#3118=DIRECTION ( 'NONE',  ( 1.000000000000000000, 0.000000000000000000, 0.000000000000000000 ) ) ;
#3123=VERTEX_POINT ( 'NONE', #12904 ) ;
#3124=LINE ( 'NONE', #1433, #16854 ) ;
#3127=CYLINDRICAL_SURFACE ( 'NONE', #8024, 1.000000000000003553 ) ;
#3134=EDGE_LOOP ( 'NONE', ( #10248, #14667 ) ) ;
#3138=VERTEX_POINT ( 'NONE', #18698 ) ;
#3148=VERTEX_POINT ( 'NONE', #300 ) ;
#3152=VERTEX_POINT ( 'NONE', #9513 ) ;
#3155=DIRECTION ( 'NONE',  ( 0.000000000000000000, 0.000000000000000000, 1.000000000000000000 ) ) ;
#3158=VECTOR ( 'NONE', #11550, 1000.000000000000000 ) ;
#3164=EDGE_CURVE ( 'NONE', #9330, #7633, #6678, .T. ) ;
#3165=DIRECTION ( 'NONE',  ( -1.000000000000000000, 0.000000000000000000, 0.000000000000000000 ) ) ;
#3166=AXIS2_PLACEMENT_3D ( 'NONE', #14478, #3856, #17668 ) ;
#3167=ORIENTED_EDGE ( 'NONE', *, *, #18231, .T. ) ;
#3172=ORIENTED_EDGE ( 'NONE', *, *, #11273, .F. ) ;
#3178=CARTESIAN_POINT ( 'NONE',  ( 5.476417968967387750, 17.43449690031536292, -35.00000000000000000 ) ) ;
#3186=CIRCLE ( 'NONE', #14381, 1.000000000000000000 ) ;
#3192=CARTESIAN_POINT ( 'NONE',  ( 8.671566133830875600, 15.77352024078954784, -35.00000000000000000 ) ) ;
#3193=FILL_AREA_STYLE_COLOUR ( '', #9941 ) ;
#3196=CARTESIAN_POINT ( 'NONE',  ( -16.11901729331276911, 5.562305898749051458, 32.00000000000000000 ) ) ;
#3212=EDGE_CURVE ( 'NONE', #12385, #15108, #3944, .T. ) ;
#3215=FACE_OUTER_BOUND ( 'NONE', #9225, .T. ) ;
#3218=AXIS2_PLACEMENT_3D ( 'NONE', #6429, #14356, #9562 ) ;
#3220=ORIENTED_EDGE ( 'NONE', *, *, #14235, .F. ) ;
#3229=ORIENTED_EDGE ( 'NONE', *, *, #4667, .T. ) ;
#3231=CIRCLE ( 'NONE', #17301, 1.000000000000004441 ) ;
#3232=DIRECTION ( 'NONE',  ( 0.000000000000000000, 0.000000000000000000, 1.000000000000000000 ) ) ;
#3237=VERTEX_POINT ( 'NONE', #6874 ) ;
#3242=VECTOR ( 'NONE', #3510, 1000.000000000000000 ) ;
#3249=VERTEX_POINT ( 'NONE', #5387 ) ;
#3250=ORIENTED_EDGE ( 'NONE', *, *, #11657, .F. ) ;
#3255=DIRECTION ( 'NONE',  ( 0.000000000000000000, 0.000000000000000000, -1.000000000000000000 ) ) ;
#3258=AXIS2_PLACEMENT_3D ( 'NONE', #17779, #5858, #19174 ) ;
#3259=AXIS2_PLACEMENT_3D ( 'NONE', #15095, #4779, #13589 ) ;
#3262=AXIS2_PLACEMENT_3D ( 'NONE', #10978, #7770, #6352 ) ;
#3264=FACE_BOUND ( 'NONE', #17721, .T. ) ;
#3266=DIRECTION ( 'NONE',  ( 0.000000000000000000, 0.000000000000000000, 1.000000000000000000 ) ) ;
#3276=CARTESIAN_POINT ( 'NONE',  ( 9.671566133830877376, 15.77352024078954784, 32.00000000000000000 ) ) ;
#3281=VECTOR ( 'NONE', #9063, 1000.000000000000000 ) ;
#3287=( GEOMETRIC_REPRESENTATION_CONTEXT ( 3 ) GLOBAL_UNCERTAINTY_ASSIGNED_CONTEXT ( ( #11595 ) ) GLOBAL_UNIT_ASSIGNED_CONTEXT ( ( #4650, #7743, #12360 ) ) REPRESENTATION_CONTEXT ( 'NONE', 'WORKASPACE' ) );
#3291=CARTESIAN_POINT ( 'NONE',  ( 3.476417968967386418, 17.43449690031536292, -35.00000000000000000 ) ) ;
#3296=DIRECTION ( 'NONE',  ( -0.000000000000000000, -0.000000000000000000, 1.000000000000000000 ) ) ;
#3304=ORIENTED_EDGE ( 'NONE', *, *, #3354, .F. ) ;
#3307=DIRECTION ( 'NONE',  ( -0.000000000000000000, -0.000000000000000000, 1.000000000000000000 ) ) ;
#3317=FACE_OUTER_BOUND ( 'NONE', #3696, .T. ) ;
#3323=ORIENTED_EDGE ( 'NONE', *, *, #3554, .F. ) ;
#3325=EDGE_LOOP ( 'NONE', ( #13310, #3374, #3961, #1678 ) ) ;
#3329=CIRCLE ( 'NONE', #3007, 1.000000000000000888 ) ;
#3331=EDGE_CURVE ( 'NONE', #15782, #8799, #14497, .T. ) ;
#3336=AXIS2_PLACEMENT_3D ( 'NONE', #8245, #5434, #6724 ) ;
#3337=EDGE_CURVE ( 'NONE', #14452, #12361, #19589, .T. ) ;
#3344=VERTEX_POINT ( 'NONE', #11690 ) ;
#3354=EDGE_CURVE ( 'NONE', #11311, #8927, #8088, .T. ) ;
#3363=VECTOR ( 'NONE', #11699, 1000.000000000000000 ) ;
#3366=DIRECTION ( 'NONE',  ( 1.000000000000000000, 0.000000000000000000, 0.000000000000000000 ) ) ;
#3367=CYLINDRICAL_SURFACE ( 'NONE', #92, 1.000000000000004441 ) ;
#3368=FACE_BOUND ( 'NONE', #13849, .T. ) ;
#3370=LINE ( 'NONE', #9482, #18442 ) ;
#3374=ORIENTED_EDGE ( 'NONE', *, *, #17291, .T. ) ;
#3378=CARTESIAN_POINT ( 'NONE',  ( 17.68117051311639898, -3.372863662543048591, -32.00000000000000000 ) ) ;
#3382=ADVANCED_FACE ( 'NONE', ( #4581, #13688, #17999, #6070, #4286, #1386, #3075, #1285, #1681, #11887, #5769, #8889, #9189, #4680, #15294, #8987, #14990, #1579, #78, #10785, #7360, #4383, #13586, #16593, #19686, #16694, #15091 ), #12092, .F. ) ;
#3387=DIRECTION ( 'NONE',  ( 0.000000000000000000, 0.000000000000000000, 1.000000000000000000 ) ) ;
#3389=VECTOR ( 'NONE', #5406, 1000.000000000000000 ) ;
#3390=ADVANCED_FACE ( 'NONE', ( #16497 ), #15389, .F. ) ;
#3396=FACE_OUTER_BOUND ( 'NONE', #12351, .T. ) ;
#3401=CARTESIAN_POINT ( 'NONE',  ( -1.255998204157475318, -17.85806462366060288, 32.00000000000000000 ) ) ;
#3405=VERTEX_POINT ( 'NONE', #13481 ) ;
#3406=CARTESIAN_POINT ( 'NONE',  ( 16.68117051311640253, -3.372863662543048591, 32.00000000000000000 ) ) ;
#3411=ORIENTED_EDGE ( 'NONE', *, *, #6990, .T. ) ;
#3413=CYLINDRICAL_SURFACE ( 'NONE', #1788, 1.000000000000004441 ) ;
#3420=CARTESIAN_POINT ( 'NONE',  ( 16.28688694438835327, -7.664027248171309203, 32.00000000000000000 ) ) ;
#3428=CARTESIAN_POINT ( 'NONE',  ( -17.96448111170888851, 1.130229351527647585, -32.00000000000000000 ) ) ;
#3430=CARTESIAN_POINT ( 'NONE',  ( 16.28688694438835327, -7.664027248171309203, -35.00000000000000000 ) ) ;
#3432=EDGE_CURVE ( 'NONE', #7344, #11827, #1175, .T. ) ;
#3434=CARTESIAN_POINT ( 'NONE',  ( 5.626241948324195441, -16.73597674598852691, 32.00000000000000000 ) ) ;
#3436=AXIS2_PLACEMENT_3D ( 'NONE', #11520, #2501, #5506 ) ;
#3451=VECTOR ( 'NONE', #7898, 1000.000000000000000 ) ;
#3456=LINE ( 'NONE', #8044, #10789 ) ;
#3468=CARTESIAN_POINT ( 'NONE',  ( -16.68117051311640253, -3.372863662543042818, 35.00000000000000000 ) ) ;
#3472=ORIENTED_EDGE ( 'NONE', *, *, #6862, .T. ) ;
#3484=EDGE_LOOP ( 'NONE', ( #4196, #9221, #8840, #10800 ) ) ;
#3487=DIRECTION ( 'NONE',  ( 1.000000000000000000, 0.000000000000000000, 0.000000000000000000 ) ) ;
#3488=VECTOR ( 'NONE', #12470, 1000.000000000000000 ) ;
#3489=DIRECTION ( 'NONE',  ( 0.000000000000000000, 0.000000000000000000, 1.000000000000000000 ) ) ;
#3501=LINE ( 'NONE', #15710, #13378 ) ;
#3505=ORIENTED_EDGE ( 'NONE', *, *, #1827, .T. ) ;
#3507=FACE_OUTER_BOUND ( 'NONE', #13416, .T. ) ;
#3510=DIRECTION ( 'NONE',  ( 0.000000000000000000, 0.000000000000000000, -1.000000000000000000 ) ) ;
#3515=EDGE_CURVE ( 'NONE', #17485, #3138, #14918, .T. ) ;
#3526=LINE ( 'NONE', #5118, #14947 ) ;
#3527=VERTEX_POINT ( 'NONE', #9338 ) ;
#3531=ADVANCED_FACE ( 'NONE', ( #9539 ), #7825, .F. ) ;
#3532=DIRECTION ( 'NONE',  ( 0.000000000000000000, 0.000000000000000000, 1.000000000000000000 ) ) ;
#3547=ORIENTED_EDGE ( 'NONE', *, *, #11666, .F. ) ;
#3554=EDGE_CURVE ( 'NONE', #15613, #15969, #8218, .T. ) ;
#3556=FACE_OUTER_BOUND ( 'NONE', #6096, .T. ) ;
#3557=AXIS2_PLACEMENT_3D ( 'NONE', #12343, #15246, #18341 ) ;
#3558=CYLINDRICAL_SURFACE ( 'NONE', #3920, 1.000000000000000888 ) ;
#3560=EDGE_CURVE ( 'NONE', #12131, #18514, #2123, .T. ) ;
#3563=LINE ( 'NONE', #9687, #15746 ) ;
#3564=EDGE_LOOP ( 'NONE', ( #18065, #15136 ) ) ;
#3567=ADVANCED_FACE ( 'NONE', ( #6606 ), #6405, .F. ) ;
#3579=CIRCLE ( 'NONE', #9023, 1.000000000000000888 ) ;
#3585=AXIS2_PLACEMENT_3D ( 'NONE', #19400, #11804, #17907 ) ;
#3586=EDGE_CURVE ( 'NONE', #11187, #11311, #14332, .T. ) ;
#3591=AXIS2_PLACEMENT_3D ( 'NONE', #13690, #3077, #15491 ) ;
#3609=ORIENTED_EDGE ( 'NONE', *, *, #7547, .T. ) ;
#3610=AXIS2_PLACEMENT_3D ( 'NONE', #1931, #14141, #8134 ) ;
#3614=VERTEX_POINT ( 'NONE', #4113 ) ;
#3628=FACE_BOUND ( 'NONE', #15050, .T. ) ;
#3629=DIRECTION ( 'NONE',  ( 0.000000000000000000, 0.000000000000000000, 1.000000000000000000 ) ) ;
#3633=CARTESIAN_POINT ( 'NONE',  ( -11.32184790671638730, 13.12143529358541549, -35.00000000000000000 ) ) ;
#3648=ORIENTED_EDGE ( 'NONE', *, *, #1885, .F. ) ;
#3653=DIRECTION ( 'NONE',  ( 1.000000000000000000, 0.000000000000000000, 0.000000000000000000 ) ) ;
#3655=EDGE_CURVE ( 'NONE', #13831, #6807, #567, .T. ) ;
#3660=FACE_BOUND ( 'NONE', #5050, .T. ) ;
#3666=EDGE_CURVE ( 'NONE', #6695, #7627, #14290, .T. ) ;
#3672=AXIS2_PLACEMENT_3D ( 'NONE', #13943, #3232, #236 ) ;
#3674=ORIENTED_EDGE ( 'NONE', *, *, #13292, .T. ) ;
#3675=DIRECTION ( 'NONE',  ( 1.000000000000000000, 0.000000000000000000, 0.000000000000000000 ) ) ;
#3677=ORIENTED_EDGE ( 'NONE', *, *, #13115, .T. ) ;
#3679=FACE_OUTER_BOUND ( 'NONE', #4476, .T. ) ;
#3687=DIRECTION ( 'NONE',  ( 0.000000000000000000, 0.000000000000000000, 1.000000000000000000 ) ) ;
#3690=VERTEX_POINT ( 'NONE', #1009 ) ;
#3696=EDGE_LOOP ( 'NONE', ( #9432, #2129, #2748, #4857 ) ) ;
#3699=ORIENTED_EDGE ( 'NONE', *, *, #6386, .T. ) ;
#3702=EDGE_CURVE ( 'NONE', #12760, #9739, #8535, .T. ) ;
#3703=DIRECTION ( 'NONE',  ( -1.000000000000000000, 0.000000000000000000, 0.000000000000000000 ) ) ;
#3704=ORIENTED_EDGE ( 'NONE', *, *, #2467, .F. ) ;
#3706=AXIS2_PLACEMENT_3D ( 'NONE', #14926, #10135, #928 ) ;
#3707=CARTESIAN_POINT ( 'NONE',  ( -14.19790265903626647, 9.644882309621941374, 32.00000000000000000 ) ) ;
#3709=DIRECTION ( 'NONE',  ( -0.000000000000000000, -0.000000000000000000, 1.000000000000000000 ) ) ;
#3712=CARTESIAN_POINT ( 'NONE',  ( 9.580134541264516912, -14.56230589874905412, 32.00000000000000000 ) ) ;
#3713=( NAMED_UNIT ( * ) PLANE_ANGLE_UNIT ( ) SI_UNIT ( $, .RADIAN. ) );
#3719=DIRECTION ( 'NONE',  ( 1.000000000000000000, 0.000000000000000000, 0.000000000000000000 ) ) ;
#3720=VECTOR ( 'NONE', #2307, 1000.000000000000000 ) ;
#3726=LINE ( 'NONE', #8228, #9649 ) ;
#3730=DIRECTION ( 'NONE',  ( 1.000000000000000000, 0.000000000000000000, 0.000000000000000000 ) ) ;
#3743=DIRECTION ( 'NONE',  ( 1.000000000000000000, 0.000000000000000000, 0.000000000000000000 ) ) ;
#3745=ORIENTED_EDGE ( 'NONE', *, *, #9552, .T. ) ;
#3748=CARTESIAN_POINT ( 'NONE',  ( -17.28688694438836393, -7.664027248171298545, 32.00000000000000000 ) ) ;
#3757=ADVANCED_FACE ( 'NONE', ( #5902 ), #10715, .F. ) ;
#3763=DIRECTION ( 'NONE',  ( 1.000000000000000000, 0.000000000000000000, 0.000000000000000000 ) ) ;
#3766=ORIENTED_EDGE ( 'NONE', *, *, #14831, .T. ) ;
#3772=VECTOR ( 'NONE', #1798, 1000.000000000000000 ) ;
#3773=CARTESIAN_POINT ( 'NONE',  ( 6.626241948324199882, -16.73597674598852691, -32.00000000000000000 ) ) ;
#3775=DIRECTION ( 'NONE',  ( 0.000000000000000000, 0.000000000000000000, 1.000000000000000000 ) ) ;
#3779=EDGE_CURVE ( 'NONE', #17931, #2783, #15894, .T. ) ;
#3784=AXIS2_PLACEMENT_3D ( 'NONE', #11665, #7237, #13362 ) ;
#3785=FACE_OUTER_BOUND ( 'NONE', #1825, .T. ) ;
#3798=ORIENTED_EDGE ( 'NONE', *, *, #14971, .F. ) ;
#3799=FACE_OUTER_BOUND ( 'NONE', #15750, .T. ) ;
#3809=ORIENTED_EDGE ( 'NONE', *, *, #18728, .F. ) ;
#3823=VERTEX_POINT ( 'NONE', #9313 ) ;
#3828=CARTESIAN_POINT ( 'NONE',  ( -12.86923836996420611, -11.47363181547641275, 32.00000000000000000 ) ) ;
#3832=CYLINDRICAL_SURFACE ( 'NONE', #4896, 1.000000000000000000 ) ;
#3833=EDGE_LOOP ( 'NONE', ( #10273, #1506 ) ) ;
#3840=CARTESIAN_POINT ( 'NONE',  ( -10.58013454126452224, -14.56230589874905235, 32.00000000000000000 ) ) ;
#3856=DIRECTION ( 'NONE',  ( -0.000000000000000000, -0.000000000000000000, 1.000000000000000000 ) ) ;
#3857=CARTESIAN_POINT ( 'NONE',  ( 9.000000000000000000, 0.000000000000000000, 29.00000000000000355 ) ) ;
#3867=DIRECTION ( 'NONE',  ( 1.000000000000000000, 0.000000000000000000, 0.000000000000000000 ) ) ;
#3874=AXIS2_PLACEMENT_3D ( 'NONE', #12938, #17632, #5226 ) ;
#3880=DIRECTION ( 'NONE',  ( 1.000000000000000000, 0.000000000000000000, 0.000000000000000000 ) ) ;
#3890=CIRCLE ( 'NONE', #14444, 1.000000000000000000 ) ;
#3898=ORIENTED_EDGE ( 'NONE', *, *, #8109, .T. ) ;
#3899=CARTESIAN_POINT ( 'NONE',  ( 9.580134541264516912, -14.56230589874905412, -32.00000000000000000 ) ) ;
#3903=CIRCLE ( 'NONE', #7395, 1.000000000000002665 ) ;
#3909=DIRECTION ( 'NONE',  ( 0.000000000000000000, 0.000000000000000000, 1.000000000000000000 ) ) ;
#3914=VERTEX_POINT ( 'NONE', #14206 ) ;
#3915=DIRECTION ( 'NONE',  ( 0.000000000000000000, 0.000000000000000000, -1.000000000000000000 ) ) ;
#3917=EDGE_CURVE ( 'NONE', #10979, #271, #13343, .T. ) ;
#3918=DIRECTION ( 'NONE',  ( 1.000000000000000000, 0.000000000000000000, 0.000000000000000000 ) ) ;
#3920=AXIS2_PLACEMENT_3D ( 'NONE', #7954, #14065, #16882 ) ;
#3921=DIRECTION ( 'NONE',  ( 1.000000000000000000, 0.000000000000000000, 0.000000000000000000 ) ) ;
#3922=ORIENTED_EDGE ( 'NONE', *, *, #13059, .T. ) ;
#3926=ADVANCED_FACE ( 'NONE', ( #6380 ), #12512, .F. ) ;
#3930=CARTESIAN_POINT ( 'NONE',  ( -17.28688694438836393, -7.664027248171298545, 35.00000000000000000 ) ) ;
#3934=CARTESIAN_POINT ( 'NONE',  ( 15.19790265903627358, 9.644882309621939598, -35.00000000000000000 ) ) ;
#3935=FACE_BOUND ( 'NONE', #6753, .T. ) ;
#3939=VERTEX_POINT ( 'NONE', #7696 ) ;
#3943=LINE ( 'NONE', #15245, #5416 ) ;
#3944=CIRCLE ( 'NONE', #5842, 1.000000000000004441 ) ;
#3948=LINE ( 'NONE', #2149, #165 ) ;
#3951=ORIENTED_EDGE ( 'NONE', *, *, #18666, .F. ) ;
#3953=DIRECTION ( 'NONE',  ( 1.000000000000000000, 0.000000000000000000, 0.000000000000000000 ) ) ;
#3956=ORIENTED_EDGE ( 'NONE', *, *, #15296, .T. ) ;
#3961=ORIENTED_EDGE ( 'NONE', *, *, #9048, .T. ) ;
#3962=DIRECTION ( 'NONE',  ( 0.000000000000000000, 0.000000000000000000, 1.000000000000000000 ) ) ;
#3969=CARTESIAN_POINT ( 'NONE',  ( -12.32184790671639085, 13.12143529358541549, 32.00000000000000000 ) ) ;
#3971=ADVANCED_FACE ( 'NONE', ( #14681 ), #8870, .F. ) ;
#3976=CARTESIAN_POINT ( 'NONE',  ( -17.11901729331276911, 5.562305898749051458, -35.00000000000000000 ) ) ;
#3987=DIRECTION ( 'NONE',  ( 0.000000000000000000, 0.000000000000000000, 1.000000000000000000 ) ) ;
#3988=VERTEX_POINT ( 'NONE', #14970 ) ;
#3990=AXIS2_PLACEMENT_3D ( 'NONE', #14854, #2635, #1151 ) ;
#3997=VERTEX_POINT ( 'NONE', #5557 ) ;
#3998=CARTESIAN_POINT ( 'NONE',  ( -12.86923836996420611, -11.47363181547641275, 32.00000000000000000 ) ) ;
#4005=VECTOR ( 'NONE', #7765, 1000.000000000000000 ) ;
#4012=ORIENTED_EDGE ( 'NONE', *, *, #18752, .T. ) ;
#4014=ORIENTED_EDGE ( 'NONE', *, *, #10919, .T. ) ;
#4015=CARTESIAN_POINT ( 'NONE',  ( -13.32184790671639618, 13.12143529358541549, -32.00000000000000000 ) ) ;
#4020=DIRECTION ( 'NONE',  ( 1.000000000000000000, 0.000000000000000000, 0.000000000000000000 ) ) ;
#4023=FACE_BOUND ( 'NONE', #17376, .T. ) ;
#4024=CYLINDRICAL_SURFACE ( 'NONE', #3706, 1.000000000000000888 ) ;
#4030=EDGE_CURVE ( 'NONE', #3614, #4548, #18561, .T. ) ;
#4035=FACE_BOUND ( 'NONE', #9481, .T. ) ;
#4036=AXIS2_PLACEMENT_3D ( 'NONE', #14828, #7100, #16327 ) ;
#4037=VERTEX_POINT ( 'NONE', #5951 ) ;
#4038=CARTESIAN_POINT ( 'NONE',  ( -17.11901729331276911, 5.562305898749051458, 35.00000000000000000 ) ) ;
#4049=CARTESIAN_POINT ( 'NONE',  ( -16.19790265903627713, 9.644882309621941374, -32.00000000000000000 ) ) ;
#4061=AXIS2_PLACEMENT_3D ( 'NONE', #13938, #4828, #10935 ) ;
#4064=EDGE_LOOP ( 'NONE', ( #4674, #4076 ) ) ;
#4066=DIRECTION ( 'NONE',  ( 0.000000000000000000, 0.000000000000000000, -1.000000000000000000 ) ) ;
#4069=CIRCLE ( 'NONE', #2800, 1.000000000000002665 ) ;
#4076=ORIENTED_EDGE ( 'NONE', *, *, #14792, .F. ) ;
#4090=AXIS2_PLACEMENT_3D ( 'NONE', #10493, #17892, #11987 ) ;
#4091=CARTESIAN_POINT ( 'NONE',  ( 8.671566133830875600, 15.77352024078954784, -32.00000000000000000 ) ) ;
#4095=CARTESIAN_POINT ( 'NONE',  ( 7.671566133830872047, 15.77352024078954784, 35.00000000000000000 ) ) ;
#4107=DIRECTION ( 'NONE',  ( 0.000000000000000000, 0.000000000000000000, 1.000000000000000000 ) ) ;
#4111=EDGE_LOOP ( 'NONE', ( #14738, #10440, #8129, #19034 ) ) ;
#4113=CARTESIAN_POINT ( 'NONE',  ( -18.68117051311639543, -3.372863662543042818, 32.00000000000000000 ) ) ;
#4116=AXIS2_PLACEMENT_3D ( 'NONE', #15043, #1042, #1332 ) ;
#4121=VERTEX_POINT ( 'NONE', #6434 ) ;
#4124=ADVANCED_FACE ( 'NONE', ( #19057 ), #11259, .F. ) ;
#4125=CARTESIAN_POINT ( 'NONE',  ( -3.255998204157480203, -17.85806462366060288, 32.00000000000000000 ) ) ;
#4127=VECTOR ( 'NONE', #9882, 1000.000000000000000 ) ;
#4128=ORIENTED_EDGE ( 'NONE', *, *, #11166, .F. ) ;
#4129=CARTESIAN_POINT ( 'NONE',  ( 9.000000000000001776, 1.102182119232617911E-15, -30.00000000000000355 ) ) ;
#4139=FILL_AREA_STYLE ('',( #3193 ) ) ;
#4140=CYLINDRICAL_SURFACE ( 'NONE', #10213, 1.000000000000002665 ) ;
#4141=DIRECTION ( 'NONE',  ( 1.000000000000000000, 0.000000000000000000, 0.000000000000000000 ) ) ;
#4151=DIRECTION ( 'NONE',  ( 0.000000000000000000, 0.000000000000000000, 1.000000000000000000 ) ) ;
#4152=CARTESIAN_POINT ( 'NONE',  ( 5.626241948324195441, -16.73597674598852691, -32.00000000000000000 ) ) ;
#4154=DIRECTION ( 'NONE',  ( 0.000000000000000000, 0.000000000000000000, 1.000000000000000000 ) ) ;
#4160=VERTEX_POINT ( 'NONE', #9668 ) ;
#4164=ORIENTED_EDGE ( 'NONE', *, *, #124, .T. ) ;
#4174=EDGE_CURVE ( 'NONE', #12336, #4629, #3456, .T. ) ;
#4195=CARTESIAN_POINT ( 'NONE',  ( 11.58013454126452579, -14.56230589874905412, 32.00000000000000000 ) ) ;
#4196=ORIENTED_EDGE ( 'NONE', *, *, #9722, .F. ) ;
#4200=LINE ( 'NONE', #718, #2936 ) ;
#4202=ORIENTED_EDGE ( 'NONE', *, *, #3779, .T. ) ;
#4209=CARTESIAN_POINT ( 'NONE',  ( -13.86923836996420967, -11.47363181547641275, 35.00000000000000000 ) ) ;
#4210=VERTEX_POINT ( 'NONE', #4049 ) ;
#4221=CIRCLE ( 'NONE', #716, 1.000000000000000888 ) ;
#4222=AXIS2_PLACEMENT_3D ( 'NONE', #18702, #2192, #16112 ) ;
#4224=DIRECTION ( 'NONE',  ( 1.000000000000000000, 0.000000000000000000, 0.000000000000000000 ) ) ;
#4226=ORIENTED_EDGE ( 'NONE', *, *, #15830, .F. ) ;
#4229=FACE_BOUND ( 'NONE', #11750, .T. ) ;
#4232=VERTEX_POINT ( 'NONE', #14661 ) ;
#4237=CIRCLE ( 'NONE', #15425, 1.000000000000004441 ) ;
#4239=CYLINDRICAL_SURFACE ( 'NONE', #8995, 1.000000000000004441 ) ;
#4242=CARTESIAN_POINT ( 'NONE',  ( 16.28688694438835327, -7.664027248171309203, -35.00000000000000000 ) ) ;
#4243=EDGE_CURVE ( 'NONE', #8143, #4160, #7575, .T. ) ;
#4249=ORIENTED_EDGE ( 'NONE', *, *, #744, .F. ) ;
#4257=VERTEX_POINT ( 'NONE', #16349 ) ;
#4263=FACE_OUTER_BOUND ( 'NONE', #19069, .T. ) ;
#4270=LINE ( 'NONE', #14778, #14132 ) ;
#4274=CARTESIAN_POINT ( 'NONE',  ( -3.255998204157480203, -17.85806462366060288, -32.00000000000000000 ) ) ;
#4275=CYLINDRICAL_SURFACE ( 'NONE', #2956, 1.000000000000000888 ) ;
#4285=DIRECTION ( 'NONE',  ( 1.000000000000000000, 0.000000000000000000, 0.000000000000000000 ) ) ;
#4286=FACE_BOUND ( 'NONE', #7271, .T. ) ;
#4291=ORIENTED_EDGE ( 'NONE', *, *, #15396, .T. ) ;
#4292=CARTESIAN_POINT ( 'NONE',  ( -9.671566133830877376, 15.77352024078954429, 35.00000000000000000 ) ) ;
#4297=DIRECTION ( 'NONE',  ( 0.000000000000000000, 0.000000000000000000, 1.000000000000000000 ) ) ;
#4300=ORIENTED_EDGE ( 'NONE', *, *, #11993, .F. ) ;
#4304=DIRECTION ( 'NONE',  ( -1.000000000000000000, 0.000000000000000000, 0.000000000000000000 ) ) ;
#4309=DIRECTION ( 'NONE',  ( -0.000000000000000000, -0.000000000000000000, 1.000000000000000000 ) ) ;
#4310=EDGE_CURVE ( 'NONE', #257, #226, #5974, .T. ) ;
#4313=DIRECTION ( 'NONE',  ( 0.000000000000000000, 0.000000000000000000, 1.000000000000000000 ) ) ;
#4315=VERTEX_POINT ( 'NONE', #2437 ) ;
#4321=CARTESIAN_POINT ( 'NONE',  ( -14.19790265903626647, 9.644882309621941374, -35.00000000000000000 ) ) ;
#4331=CARTESIAN_POINT ( 'NONE',  ( 10.58013454126452046, -14.56230589874905412, 35.00000000000000000 ) ) ;
#4349=DIRECTION ( 'NONE',  ( -0.000000000000000000, -0.000000000000000000, 1.000000000000000000 ) ) ;
#4363=CARTESIAN_POINT ( 'NONE',  ( 5.510910596163084625E-16, 18.00000000000000355, -32.00000000000000000 ) ) ;
#4368=ORIENTED_EDGE ( 'NONE', *, *, #1066, .T. ) ;
#4369=DIRECTION ( 'NONE',  ( 1.000000000000000000, 0.000000000000000000, 0.000000000000000000 ) ) ;
#4383=FACE_BOUND ( 'NONE', #1657, .T. ) ;
#4392=ORIENTED_EDGE ( 'NONE', *, *, #10326, .T. ) ;
#4393=DIRECTION ( 'NONE',  ( 0.000000000000000000, 0.000000000000000000, 1.000000000000000000 ) ) ;
#4407=DIRECTION ( 'NONE',  ( -1.000000000000000000, 0.000000000000000000, 0.000000000000000000 ) ) ;
#4415=AXIS2_PLACEMENT_3D ( 'NONE', #13094, #17695, #18093 ) ;
#4423=DIRECTION ( 'NONE',  ( 0.000000000000000000, 0.000000000000000000, -1.000000000000000000 ) ) ;
#4426=DIRECTION ( 'NONE',  ( -1.000000000000000000, 0.000000000000000000, 0.000000000000000000 ) ) ;
#4434=EDGE_CURVE ( 'NONE', #18092, #1561, #3526, .T. ) ;
#4435=CARTESIAN_POINT ( 'NONE',  ( 8.671566133830875600, 15.77352024078954784, 35.00000000000000000 ) ) ;
#4436=CARTESIAN_POINT ( 'NONE',  ( 8.671566133830875600, 15.77352024078954784, 32.00000000000000000 ) ) ;
#4444=EDGE_LOOP ( 'NONE', ( #11937, #7019 ) ) ;
#4445=CARTESIAN_POINT ( 'NONE',  ( -14.00000000000000178, 0.000000000000000000, 35.00000000000000000 ) ) ;
#4448=DIRECTION ( 'NONE',  ( 0.000000000000000000, 0.000000000000000000, -1.000000000000000000 ) ) ;
#4450=CARTESIAN_POINT ( 'NONE',  ( -14.86923836996421144, -11.47363181547641275, -32.00000000000000000 ) ) ;
#4452=ORIENTED_EDGE ( 'NONE', *, *, #1066, .F. ) ;
#4454=ORIENTED_EDGE ( 'NONE', *, *, #17752, .F. ) ;
#4459=VERTEX_POINT ( 'NONE', #18730 ) ;
#4460=ORIENTED_EDGE ( 'NONE', *, *, #3164, .T. ) ;
#4471=LINE ( 'NONE', #10583, #15160 ) ;
#4474=CIRCLE ( 'NONE', #1280, 12.00000000000000178 ) ;
#4476=EDGE_LOOP ( 'NONE', ( #4651, #2073, #218, #5103 ) ) ;
#4477=CYLINDRICAL_SURFACE ( 'NONE', #6626, 0.9999999999999974465 ) ;
#4489=CARTESIAN_POINT ( 'NONE',  ( -14.00000000000000178, 0.000000000000000000, 32.00000000000000000 ) ) ;
#4496=CARTESIAN_POINT ( 'NONE',  ( -17.68117051311639898, -3.372863662543042818, 32.00000000000000000 ) ) ;
#4501=DIRECTION ( 'NONE',  ( 0.000000000000000000, 0.000000000000000000, 1.000000000000000000 ) ) ;
#4502=DIRECTION ( 'NONE',  ( -0.000000000000000000, -0.000000000000000000, 1.000000000000000000 ) ) ;
#4507=VERTEX_POINT ( 'NONE', #5417 ) ;
#4518=EDGE_CURVE ( 'NONE', #11655, #4548, #16235, .T. ) ;
#4521=EDGE_CURVE ( 'NONE', #3152, #18644, #6300, .T. ) ;
#4526=DIRECTION ( 'NONE',  ( 0.000000000000000000, 0.000000000000000000, -1.000000000000000000 ) ) ;
#4529=AXIS2_PLACEMENT_3D ( 'NONE', #10139, #19423, #16237 ) ;
#4532=EDGE_LOOP ( 'NONE', ( #1737, #3250, #8557, #3766 ) ) ;
#4533=CIRCLE ( 'NONE', #10609, 1.000000000000004441 ) ;
#4546=AXIS2_PLACEMENT_3D ( 'NONE', #7777, #183, #277 ) ;
#4547=CYLINDRICAL_SURFACE ( 'NONE', #10342, 1.000000000000003109 ) ;
#4548=VERTEX_POINT ( 'NONE', #10230 ) ;
#4559=ORIENTED_EDGE ( 'NONE', *, *, #4243, .F. ) ;
#4560=EDGE_CURVE ( 'NONE', #12621, #18193, #1851, .T. ) ;
#4562=CARTESIAN_POINT ( 'NONE',  ( 15.19790265903627358, 9.644882309621939598, 32.00000000000000000 ) ) ;
#4563=VERTEX_POINT ( 'NONE', #8619 ) ;
#4567=AXIS2_PLACEMENT_3D ( 'NONE', #1642, #7735, #8951 ) ;
#4572=CARTESIAN_POINT ( 'NONE',  ( 0.000000000000000000, 0.000000000000000000, 35.00000000000000000 ) ) ;
#4573=ADVANCED_FACE ( 'NONE', ( #10041 ), #2605, .F. ) ;
#4581=FACE_BOUND ( 'NONE', #7700, .T. ) ;
#4584=CARTESIAN_POINT ( 'NONE',  ( 12.86923836996420967, -11.47363181547641453, 32.00000000000000000 ) ) ;
#4587=DIRECTION ( 'NONE',  ( 1.000000000000000000, 0.000000000000000000, 0.000000000000000000 ) ) ;
#4596=DIRECTION ( 'NONE',  ( 0.000000000000000000, 0.000000000000000000, -1.000000000000000000 ) ) ;
#4599=EDGE_CURVE ( 'NONE', #9729, #19421, #1220, .T. ) ;
#4602=DIRECTION ( 'NONE',  ( -1.000000000000000000, 0.000000000000000000, 0.000000000000000000 ) ) ;
#4622=CARTESIAN_POINT ( 'NONE',  ( 14.86923836996420434, -11.47363181547641453, -35.00000000000000000 ) ) ;
#4624=AXIS2_PLACEMENT_3D ( 'NONE', #6087, #3094, #12010 ) ;
#4626=CARTESIAN_POINT ( 'NONE',  ( -4.476417968967385974, 17.43449690031536292, -32.00000000000000000 ) ) ;
#4629=VERTEX_POINT ( 'NONE', #10718 ) ;
#4635=ORIENTED_EDGE ( 'NONE', *, *, #2705, .F. ) ;
#4637=EDGE_CURVE ( 'NONE', #19430, #18625, #19422, .T. ) ;
#4639=ADVANCED_FACE ( 'NONE', ( #15120 ), #1213, .F. ) ;
#4640=ORIENTED_EDGE ( 'NONE', *, *, #12744, .F. ) ;
#4650=( LENGTH_UNIT ( ) NAMED_UNIT ( * ) SI_UNIT ( .MILLI., .METRE. ) );
#4651=ORIENTED_EDGE ( 'NONE', *, *, #12165, .F. ) ;
#4659=VERTEX_POINT ( 'NONE', #14923 ) ;
#4663=CIRCLE ( 'NONE', #16494, 0.9999999999999974465 ) ;
#4667=EDGE_CURVE ( 'NONE', #18721, #3997, #5800, .T. ) ;
#4672=AXIS2_PLACEMENT_3D ( 'NONE', #10344, #4423, #15132 ) ;
#4674=ORIENTED_EDGE ( 'NONE', *, *, #12667, .F. ) ;
#4680=FACE_BOUND ( 'NONE', #8208, .T. ) ;
#4682=EDGE_CURVE ( 'NONE', #9602, #12131, #9526, .T. ) ;
#4683=LINE ( 'NONE', #10984, #16378 ) ;
#4692=EDGE_CURVE ( 'NONE', #10790, #12820, #9211, .T. ) ;
#4694=CARTESIAN_POINT ( 'NONE',  ( 17.68117051311639898, -3.372863662543048591, -35.00000000000000000 ) ) ;
#4696=DIRECTION ( 'NONE',  ( 0.000000000000000000, 0.000000000000000000, -1.000000000000000000 ) ) ;
#4707=EDGE_LOOP ( 'NONE', ( #2395, #2145 ) ) ;
#4717=AXIS2_PLACEMENT_3D ( 'NONE', #18605, #18411, #11006 ) ;
#4720=ORIENTED_EDGE ( 'NONE', *, *, #10864, .F. ) ;
#4725=ORIENTED_EDGE ( 'NONE', *, *, #18116, .F. ) ;
#4727=VERTEX_POINT ( 'NONE', #16726 ) ;
#4728=CARTESIAN_POINT ( 'NONE',  ( -13.86923836996420967, -11.47363181547641275, -35.00000000000000000 ) ) ;
#4731=CIRCLE ( 'NONE', #4090, 0.9999999999999974465 ) ;
#4733=AXIS2_PLACEMENT_3D ( 'NONE', #12121, #4502, #10619 ) ;
#4734=EDGE_LOOP ( 'NONE', ( #12024, #15867, #5531, #17461 ) ) ;
#4736=EDGE_CURVE ( 'NONE', #2023, #12048, #3004, .T. ) ;
#4740=VECTOR ( 'NONE', #11767, 1000.000000000000000 ) ;
#4750=VERTEX_POINT ( 'NONE', #17117 ) ;
#4751=EDGE_CURVE ( 'NONE', #11811, #3123, #9615, .T. ) ;
#4752=ORIENTED_EDGE ( 'NONE', *, *, #10327, .F. ) ;
#4753=CARTESIAN_POINT ( 'NONE',  ( -16.28688694438836038, -7.664027248171298545, 32.00000000000000000 ) ) ;
#4757=EDGE_CURVE ( 'NONE', #17855, #17528, #11118, .T. ) ;
#4763=CARTESIAN_POINT ( 'NONE',  ( 7.626241948324204323, -16.73597674598852691, -32.00000000000000000 ) ) ;
#4764=FACE_OUTER_BOUND ( 'NONE', #16120, .T. ) ;
#4778=DIRECTION ( 'NONE',  ( 0.000000000000000000, 0.000000000000000000, 1.000000000000000000 ) ) ;
#4779=DIRECTION ( 'NONE',  ( 0.000000000000000000, 0.000000000000000000, -1.000000000000000000 ) ) ;
#4786=ORIENTED_EDGE ( 'NONE', *, *, #16300, .F. ) ;
#4798=EDGE_LOOP ( 'NONE', ( #14567, #512, #16554, #435 ) ) ;
#4817=EDGE_LOOP ( 'NONE', ( #16060, #3898, #15471, #9741 ) ) ;
#4818=VECTOR ( 'NONE', #10658, 1000.000000000000000 ) ;
#4820=FACE_OUTER_BOUND ( 'NONE', #1045, .T. ) ;
#4821=ORIENTED_EDGE ( 'NONE', *, *, #11779, .F. ) ;
#4822=CYLINDRICAL_SURFACE ( 'NONE', #9598, 1.000000000000002665 ) ;
#4828=DIRECTION ( 'NONE',  ( 0.000000000000000000, 0.000000000000000000, 1.000000000000000000 ) ) ;
#4829=DIRECTION ( 'NONE',  ( 1.000000000000000000, 0.000000000000000000, 0.000000000000000000 ) ) ;
#4830=ORIENTED_EDGE ( 'NONE', *, *, #3012, .T. ) ;
#4832=CIRCLE ( 'NONE', #10270, 1.000000000000000888 ) ;
#4834=AXIS2_PLACEMENT_3D ( 'NONE', #538, #2318, #3918 ) ;
#4836=EDGE_CURVE ( 'NONE', #3344, #4257, #16925, .T. ) ;
#4850=EDGE_CURVE ( 'NONE', #676, #19176, #7923, .T. ) ;
#4852=AXIS2_PLACEMENT_3D ( 'NONE', #6196, #9219, #6382 ) ;
#4854=EDGE_LOOP ( 'NONE', ( #16505, #8222, #18963, #15871 ) ) ;
#4857=ORIENTED_EDGE ( 'NONE', *, *, #18421, .F. ) ;
#4859=CARTESIAN_POINT ( 'NONE',  ( -17.11901729331276911, 5.562305898749051458, -32.00000000000000000 ) ) ;
#4866=CARTESIAN_POINT ( 'NONE',  ( 7.626241948324204323, -16.73597674598852691, 32.00000000000000000 ) ) ;
#4867=CARTESIAN_POINT ( 'NONE',  ( -11.58013454126452579, -14.56230589874905235, 35.00000000000000000 ) ) ;
#4868=ORIENTED_EDGE ( 'NONE', *, *, #14971, .T. ) ;
#4875=AXIS2_PLACEMENT_3D ( 'NONE', #1079, #7154, #13280 ) ;
#4879=DIRECTION ( 'NONE',  ( 1.000000000000000000, 0.000000000000000000, 0.000000000000000000 ) ) ;
#4883=CARTESIAN_POINT ( 'NONE',  ( -13.86923836996420967, -11.47363181547641275, -35.00000000000000000 ) ) ;
#4886=CARTESIAN_POINT ( 'NONE',  ( 4.476417968967386862, 17.43449690031536292, -32.00000000000000000 ) ) ;
#4888=CARTESIAN_POINT ( 'NONE',  ( 12.86923836996420967, -11.47363181547641453, -35.00000000000000000 ) ) ;
#4891=DIRECTION ( 'NONE',  ( 1.000000000000000000, 0.000000000000000000, 0.000000000000000000 ) ) ;
#4896=AXIS2_PLACEMENT_3D ( 'NONE', #19136, #17640, #932 ) ;
#4902=ORIENTED_EDGE ( 'NONE', *, *, #5649, .T. ) ;
#4909=ORIENTED_EDGE ( 'NONE', *, *, #17852, .T. ) ;
#4910=CARTESIAN_POINT ( 'NONE',  ( 12.00000000000000178, 1.469576158976824144E-15, -30.00000000000000355 ) ) ;
#4912=VERTEX_POINT ( 'NONE', #4095 ) ;
#4915=DIRECTION ( 'NONE',  ( 1.000000000000000000, 0.000000000000000000, 0.000000000000000000 ) ) ;
#4926=ADVANCED_FACE ( 'NONE', ( #12096 ), #2777, .T. ) ;
#4930=DIRECTION ( 'NONE',  ( -1.000000000000000000, 0.000000000000000000, 0.000000000000000000 ) ) ;
#4956=EDGE_LOOP ( 'NONE', ( #4902, #11031 ) ) ;
#4968=ORIENTED_EDGE ( 'NONE', *, *, #8826, .T. ) ;
#4975=AXIS2_PLACEMENT_3D ( 'NONE', #2458, #5165, #14494 ) ;
#4976=DIRECTION ( 'NONE',  ( 0.000000000000000000, 0.000000000000000000, 1.000000000000000000 ) ) ;
#4979=CARTESIAN_POINT ( 'NONE',  ( 22.00000000000000355, 0.000000000000000000, 32.00000000000000000 ) ) ;
#4982=EDGE_CURVE ( 'NONE', #9521, #9108, #10593, .T. ) ;
#4984=CIRCLE ( 'NONE', #1787, 1.000000000000000888 ) ;
#4986=DIRECTION ( 'NONE',  ( 0.000000000000000000, 0.000000000000000000, -1.000000000000000000 ) ) ;
#4992=FACE_OUTER_BOUND ( 'NONE', #15582, .T. ) ;
#4993=PRESENTATION_STYLE_ASSIGNMENT (( #9509 ) ) ;
#4994=EDGE_LOOP ( 'NONE', ( #961, #14263 ) ) ;
#5000=EDGE_CURVE ( 'NONE', #8773, #11695, #13788, .T. ) ;
#5004=DIRECTION ( 'NONE',  ( 1.000000000000000000, 0.000000000000000000, 0.000000000000000000 ) ) ;
#5008=ORIENTED_EDGE ( 'NONE', *, *, #1840, .T. ) ;
#5011=CARTESIAN_POINT ( 'NONE',  ( 22.00000000000000355, 0.000000000000000000, 35.00000000000000000 ) ) ;
#5013=CARTESIAN_POINT ( 'NONE',  ( 8.671566133830875600, 15.77352024078954784, -32.00000000000000000 ) ) ;
#5014=LINE ( 'NONE', #15825, #19577 ) ;
#5015=DIRECTION ( 'NONE',  ( -0.000000000000000000, -0.000000000000000000, -1.000000000000000000 ) ) ;
#5027=EDGE_LOOP ( 'NONE', ( #16340, #9939, #15904, #19026 ) ) ;
#5033=AXIS2_PLACEMENT_3D ( 'NONE', #4242, #949, #11463 ) ;
#5035=LINE ( 'NONE', #3828, #10957 ) ;
#5036=DIRECTION ( 'NONE',  ( 0.000000000000000000, 0.000000000000000000, -1.000000000000000000 ) ) ;
#5042=LINE ( 'NONE', #557, #2373 ) ;
#5043=AXIS2_PLACEMENT_3D ( 'NONE', #18999, #14604, #984 ) ;
#5050=EDGE_LOOP ( 'NONE', ( #16432, #11286 ) ) ;
#5051=DIRECTION ( 'NONE',  ( 1.000000000000000000, 0.000000000000000000, 0.000000000000000000 ) ) ;
#5056=VECTOR ( 'NONE', #17281, 1000.000000000000000 ) ;
#5060=FACE_OUTER_BOUND ( 'NONE', #2535, .T. ) ;
#5061=FACE_BOUND ( 'NONE', #14803, .T. ) ;
#5071=PRODUCT_DEFINITION_FORMATION_WITH_SPECIFIED_SOURCE ( 'ANY', '', #17368, .NOT_KNOWN. ) ;
#5078=AXIS2_PLACEMENT_3D ( 'NONE', #10165, #17569, #3763 ) ;
#5080=DIRECTION ( 'NONE',  ( 0.000000000000000000, 0.000000000000000000, -1.000000000000000000 ) ) ;
#5086=ORIENTED_EDGE ( 'NONE', *, *, #14648, .F. ) ;
#5099=ORIENTED_EDGE ( 'NONE', *, *, #10121, .T. ) ;
#5100=EDGE_CURVE ( 'NONE', #13272, #9559, #8804, .T. ) ;
#5103=ORIENTED_EDGE ( 'NONE', *, *, #11112, .F. ) ;
#5105=DIRECTION ( 'NONE',  ( -1.000000000000000000, 0.000000000000000000, 0.000000000000000000 ) ) ;
#5111=ORIENTED_EDGE ( 'NONE', *, *, #13538, .F. ) ;
#5112=AXIS2_PLACEMENT_3D ( 'NONE', #12802, #8402, #8198 ) ;
#5115=EDGE_CURVE ( 'NONE', #16011, #8576, #2272, .T. ) ;
#5118=CARTESIAN_POINT ( 'NONE',  ( 14.86923836996420434, -11.47363181547641453, -32.00000000000000000 ) ) ;
#5119=EDGE_LOOP ( 'NONE', ( #11179, #13248, #11514, #13307 ) ) ;
#5120=DIRECTION ( 'NONE',  ( 0.000000000000000000, 0.000000000000000000, 1.000000000000000000 ) ) ;
#5126=CARTESIAN_POINT ( 'NONE',  ( 6.626241948324199882, -16.73597674598852691, -35.00000000000000000 ) ) ;
#5129=ORIENTED_EDGE ( 'NONE', *, *, #10628, .F. ) ;
#5135=EDGE_CURVE ( 'NONE', #10068, #3527, #2088, .T. ) ;
#5148=CIRCLE ( 'NONE', #5786, 1.000000000000000888 ) ;
#5153=FACE_BOUND ( 'NONE', #6399, .T. ) ;
#5160=ORIENTED_EDGE ( 'NONE', *, *, #1632, .T. ) ;
#5165=DIRECTION ( 'NONE',  ( 0.000000000000000000, 0.000000000000000000, 1.000000000000000000 ) ) ;
#5166=CIRCLE ( 'NONE', #15092, 1.000000000000002665 ) ;
#5168=ADVANCED_FACE ( 'NONE', ( #5561 ), #12883, .F. ) ;
#5170=AXIS2_PLACEMENT_3D ( 'NONE', #18831, #11339, #8127 ) ;
#5171=DIRECTION ( 'NONE',  ( -0.000000000000000000, -0.000000000000000000, 1.000000000000000000 ) ) ;
#5172=VERTEX_POINT ( 'NONE', #11671 ) ;
#5173=DIRECTION ( 'NONE',  ( 0.000000000000000000, 0.000000000000000000, 1.000000000000000000 ) ) ;
#5175=EDGE_CURVE ( 'NONE', #11476, #3823, #11371, .T. ) ;
#5184=CIRCLE ( 'NONE', #15426, 1.000000000000002665 ) ;
#5185=CARTESIAN_POINT ( 'NONE',  ( -9.671566133830877376, 15.77352024078954429, 32.00000000000000000 ) ) ;
#5186=EDGE_LOOP ( 'NONE', ( #16500, #5213, #7235, #4300 ) ) ;
#5187=DIRECTION ( 'NONE',  ( 0.000000000000000000, 0.000000000000000000, 1.000000000000000000 ) ) ;
#5191=CARTESIAN_POINT ( 'NONE',  ( 12.32184790671639618, 13.12143529358541016, -32.00000000000000000 ) ) ;
#5196=ORIENTED_EDGE ( 'NONE', *, *, #13088, .T. ) ;
#5198=EDGE_CURVE ( 'NONE', #16569, #16271, #15839, .T. ) ;
#5206=EDGE_CURVE ( 'NONE', #2023, #13547, #12329, .T. ) ;
#5211=LINE ( 'NONE', #17619, #3720 ) ;
#5213=ORIENTED_EDGE ( 'NONE', *, *, #13583, .T. ) ;
#5215=ORIENTED_EDGE ( 'NONE', *, *, #3586, .T. ) ;
#5222=LINE ( 'NONE', #9641, #15720 ) ;
#5224=ORIENTED_EDGE ( 'NONE', *, *, #3655, .T. ) ;
#5226=DIRECTION ( 'NONE',  ( 1.000000000000000000, 0.000000000000000000, -0.000000000000000000 ) ) ;
#5232=CARTESIAN_POINT ( 'NONE',  ( 5.626241948324195441, -16.73597674598852691, -32.00000000000000000 ) ) ;
#5240=CYLINDRICAL_SURFACE ( 'NONE', #13557, 1.000000000000002665 ) ;
#5244=CARTESIAN_POINT ( 'NONE',  ( 18.68117051311639543, -3.372863662543048591, 32.00000000000000000 ) ) ;
#5249=CARTESIAN_POINT ( 'NONE',  ( 17.68117051311639898, -3.372863662543048591, 32.00000000000000000 ) ) ;
#5255=ORIENTED_EDGE ( 'NONE', *, *, #9270, .T. ) ;
#5260=CARTESIAN_POINT ( 'NONE',  ( -2.255998204157477538, -17.85806462366060288, -32.00000000000000000 ) ) ;
#5261=EDGE_LOOP ( 'NONE', ( #15884, #7933 ) ) ;
#5262=DIRECTION ( 'NONE',  ( 0.000000000000000000, 0.000000000000000000, 1.000000000000000000 ) ) ;
#5264=DIRECTION ( 'NONE',  ( 0.000000000000000000, 0.000000000000000000, -1.000000000000000000 ) ) ;
#5271=AXIS2_PLACEMENT_3D ( 'NONE', #7876, #3387, #15595 ) ;
#5292=ADVANCED_FACE ( 'NONE', ( #7146 ), #7242, .F. ) ;
#5294=DIRECTION ( 'NONE',  ( 0.000000000000000000, 0.000000000000000000, 1.000000000000000000 ) ) ;
#5305=VERTEX_POINT ( 'NONE', #18076 ) ;
#5311=CARTESIAN_POINT ( 'NONE',  ( 16.11901729331276556, 5.562305898749055011, -32.00000000000000000 ) ) ;
#5313=VERTEX_POINT ( 'NONE', #10477 ) ;
#5315=ORIENTED_EDGE ( 'NONE', *, *, #14959, .F. ) ;
#5316=DIRECTION ( 'NONE',  ( 1.000000000000000000, 0.000000000000000000, 0.000000000000000000 ) ) ;
#5320=AXIS2_PLACEMENT_3D ( 'NONE', #10891, #14286, #9292 ) ;
#5325=FACE_BOUND ( 'NONE', #11568, .T. ) ;
#5326=CYLINDRICAL_SURFACE ( 'NONE', #5607, 0.9999999999999974465 ) ;
#5328=AXIS2_PLACEMENT_3D ( 'NONE', #390, #9209, #15311 ) ;
#5329=DIRECTION ( 'NONE',  ( -1.000000000000000000, 0.000000000000000000, 0.000000000000000000 ) ) ;
#5330=AXIS2_PLACEMENT_3D ( 'NONE', #1604, #6578, #205 ) ;
#5333=ORIENTED_EDGE ( 'NONE', *, *, #18231, .F. ) ;
#5337=ORIENTED_EDGE ( 'NONE', *, *, #3702, .T. ) ;
#5340=CARTESIAN_POINT ( 'NONE',  ( -11.32184790671638730, 13.12143529358541549, -32.00000000000000000 ) ) ;
#5354=CARTESIAN_POINT ( 'NONE',  ( -15.28688694438835505, -7.664027248171298545, -32.00000000000000000 ) ) ;
#5369=ORIENTED_EDGE ( 'NONE', *, *, #9301, .F. ) ;
#5372=ORIENTED_EDGE ( 'NONE', *, *, #10549, .F. ) ;
#5379=ADVANCED_FACE ( 'NONE', ( #17239 ), #9645, .F. ) ;
#5385=CARTESIAN_POINT ( 'NONE',  ( 4.476417968967386862, 17.43449690031536292, 32.00000000000000000 ) ) ;
#5387=CARTESIAN_POINT ( 'NONE',  ( 17.28688694438834972, -7.664027248171309203, 35.00000000000000000 ) ) ;
#5397=DIRECTION ( 'NONE',  ( 0.000000000000000000, 0.000000000000000000, 1.000000000000000000 ) ) ;
#5401=ADVANCED_FACE ( 'NONE', ( #14137 ), #5326, .F. ) ;
#5405=ORIENTED_EDGE ( 'NONE', *, *, #8309, .F. ) ;
#5406=DIRECTION ( 'NONE',  ( 0.000000000000000000, 0.000000000000000000, -1.000000000000000000 ) ) ;
#5415=DIRECTION ( 'NONE',  ( -0.000000000000000000, -0.000000000000000000, 1.000000000000000000 ) ) ;
#5416=VECTOR ( 'NONE', #18050, 1000.000000000000000 ) ;
#5417=CARTESIAN_POINT ( 'NONE',  ( -12.00000000000000178, 0.000000000000000000, -30.00000000000000355 ) ) ;
#5419=FACE_BOUND ( 'NONE', #7383, .T. ) ;
#5420=DIRECTION ( 'NONE',  ( 0.000000000000000000, 0.000000000000000000, 1.000000000000000000 ) ) ;
#5422=EDGE_CURVE ( 'NONE', #18804, #8859, #2106, .T. ) ;
#5434=DIRECTION ( 'NONE',  ( -0.000000000000000000, -0.000000000000000000, 1.000000000000000000 ) ) ;
#5439=DIRECTION ( 'NONE',  ( 1.000000000000000000, 0.000000000000000000, 0.000000000000000000 ) ) ;
#5440=ORIENTED_EDGE ( 'NONE', *, *, #11529, .F. ) ;
#5441=DIRECTION ( 'NONE',  ( 1.000000000000000000, 0.000000000000000000, 0.000000000000000000 ) ) ;
#5454=ORIENTED_EDGE ( 'NONE', *, *, #14648, .T. ) ;
#5457=ORIENTED_EDGE ( 'NONE', *, *, #8478, .T. ) ;
#5460=DIRECTION ( 'NONE',  ( 0.000000000000000000, 0.000000000000000000, -1.000000000000000000 ) ) ;
#5463=DIRECTION ( 'NONE',  ( 1.000000000000000000, 0.000000000000000000, 0.000000000000000000 ) ) ;
#5480=CIRCLE ( 'NONE', #13161, 1.000000000000002665 ) ;
#5494=VECTOR ( 'NONE', #6082, 1000.000000000000000 ) ;
#5495=AXIS2_PLACEMENT_3D ( 'NONE', #16190, #13276, #11773 ) ;
#5506=DIRECTION ( 'NONE',  ( 1.000000000000000000, 0.000000000000000000, 0.000000000000000000 ) ) ;
#5507=ORIENTED_EDGE ( 'NONE', *, *, #17312, .F. ) ;
#5508=DIRECTION ( 'NONE',  ( 0.000000000000000000, 0.000000000000000000, 1.000000000000000000 ) ) ;
#5514=AXIS2_PLACEMENT_3D ( 'NONE', #15940, #2223, #10134 ) ;
#5516=CARTESIAN_POINT ( 'NONE',  ( 0.000000000000000000, 0.000000000000000000, -30.00000000000000355 ) ) ;
#5517=EDGE_LOOP ( 'NONE', ( #12064, #12264 ) ) ;
#5530=DIRECTION ( 'NONE',  ( 1.000000000000000000, 0.000000000000000000, 0.000000000000000000 ) ) ;
#5531=ORIENTED_EDGE ( 'NONE', *, *, #17001, .T. ) ;
#5543=EDGE_CURVE ( 'NONE', #1207, #3249, #5933, .T. ) ;
#5544=DIRECTION ( 'NONE',  ( 0.000000000000000000, 0.000000000000000000, 1.000000000000000000 ) ) ;
#5553=ADVANCED_FACE ( 'NONE', ( #16431 ), #4024, .F. ) ;
#5557=CARTESIAN_POINT ( 'NONE',  ( 13.32184790671640151, 13.12143529358541016, -35.00000000000000000 ) ) ;
#5558=AXIS2_PLACEMENT_3D ( 'NONE', #2181, #8286, #14398 ) ;
#5559=ORIENTED_EDGE ( 'NONE', *, *, #11628, .T. ) ;
#5561=FACE_OUTER_BOUND ( 'NONE', #14868, .T. ) ;
#5564=DIRECTION ( 'NONE',  ( 0.000000000000000000, 0.000000000000000000, 1.000000000000000000 ) ) ;
#5566=VERTEX_POINT ( 'NONE', #13130 ) ;
#5575=CARTESIAN_POINT ( 'NONE',  ( 16.96448111170888851, 1.130229351527639370, 35.00000000000000000 ) ) ;
#5596=EDGE_CURVE ( 'NONE', #17754, #1977, #12670, .T. ) ;
#5599=DIRECTION ( 'NONE',  ( -0.000000000000000000, -0.000000000000000000, 1.000000000000000000 ) ) ;
#5607=AXIS2_PLACEMENT_3D ( 'NONE', #8131, #3629, #3730 ) ;
#5614=ORIENTED_EDGE ( 'NONE', *, *, #3655, .F. ) ;
#5631=DIRECTION ( 'NONE',  ( 0.000000000000000000, 0.000000000000000000, 1.000000000000000000 ) ) ;
#5632=EDGE_CURVE ( 'NONE', #4257, #13799, #6566, .T. ) ;
#5639=CARTESIAN_POINT ( 'NONE',  ( 4.476417968967386862, 17.43449690031536292, 35.00000000000000000 ) ) ;
#5643=EDGE_CURVE ( 'NONE', #11476, #2678, #17633, .T. ) ;
#5649=EDGE_CURVE ( 'NONE', #12547, #14379, #17774, .T. ) ;
#5651=AXIS2_PLACEMENT_3D ( 'NONE', #7919, #1732, #6313 ) ;
#5654=CARTESIAN_POINT ( 'NONE',  ( -3.476417968967383754, 17.43449690031536292, -32.00000000000000000 ) ) ;
#5660=FACE_OUTER_BOUND ( 'NONE', #11420, .T. ) ;
#5679=CARTESIAN_POINT ( 'NONE',  ( -16.96448111170888851, 1.130229351527647585, 32.00000000000000000 ) ) ;
#5680=ORIENTED_EDGE ( 'NONE', *, *, #662, .T. ) ;
#5687=AXIS2_PLACEMENT_3D ( 'NONE', #11381, #7042, #12071 ) ;
#5698=FACE_OUTER_BOUND ( 'NONE', #9534, .T. ) ;
#5704=ORIENTED_EDGE ( 'NONE', *, *, #13766, .F. ) ;
#5705=DIRECTION ( 'NONE',  ( 0.000000000000000000, 0.000000000000000000, -1.000000000000000000 ) ) ;
#5711=VERTEX_POINT ( 'NONE', #7604 ) ;
#5720=CYLINDRICAL_SURFACE ( 'NONE', #6915, 9.000000000000000000 ) ;
#5728=ORIENTED_EDGE ( 'NONE', *, *, #5135, .F. ) ;
#5734=CIRCLE ( 'NONE', #8308, 1.000000000000004441 ) ;
#5735=DIRECTION ( 'NONE',  ( 1.000000000000000000, 0.000000000000000000, 0.000000000000000000 ) ) ;
#5738=DIRECTION ( 'NONE',  ( 1.000000000000000000, 0.000000000000000000, 0.000000000000000000 ) ) ;
#5740=VERTEX_POINT ( 'NONE', #7501 ) ;
#5742=EDGE_LOOP ( 'NONE', ( #16268, #6360 ) ) ;
#5744=DIRECTION ( 'NONE',  ( 1.000000000000000000, 0.000000000000000000, 0.000000000000000000 ) ) ;
#5751=ORIENTED_EDGE ( 'NONE', *, *, #3212, .F. ) ;
#5753=VERTEX_POINT ( 'NONE', #9319 ) ;
#5758=AXIS2_PLACEMENT_3D ( 'NONE', #15155, #15056, #1348 ) ;
#5759=AXIS2_PLACEMENT_3D ( 'NONE', #15270, #6144, #12263 ) ;
#5769=FACE_BOUND ( 'NONE', #19427, .T. ) ;
#5775=ORIENTED_EDGE ( 'NONE', *, *, #8109, .F. ) ;
#5777=CIRCLE ( 'NONE', #3557, 1.000000000000000888 ) ;
#5785=EDGE_LOOP ( 'NONE', ( #18529, #17223 ) ) ;
#5786=AXIS2_PLACEMENT_3D ( 'NONE', #8725, #8443, #17639 ) ;
#5787=AXIS2_PLACEMENT_3D ( 'NONE', #19595, #8598, #1194 ) ;
#5791=ORIENTED_EDGE ( 'NONE', *, *, #1143, .F. ) ;
#5793=ORIENTED_EDGE ( 'NONE', *, *, #6862, .F. ) ;
#5795=CARTESIAN_POINT ( 'NONE',  ( -1.000000000000001998, 18.00000000000000355, -32.00000000000000000 ) ) ;
#5800=LINE ( 'NONE', #16526, #10805 ) ;
#5801=EDGE_LOOP ( 'NONE', ( #1409, #1564, #7140, #11046 ) ) ;
#5804=EDGE_CURVE ( 'NONE', #17520, #15780, #4663, .T. ) ;
#5807=AXIS2_PLACEMENT_3D ( 'NONE', #6762, #9897, #1268 ) ;
#5811=ORIENTED_EDGE ( 'NONE', *, *, #17071, .F. ) ;
#5815=FACE_BOUND ( 'NONE', #8607, .T. ) ;
#5817=DIRECTION ( 'NONE',  ( 1.000000000000000000, 0.000000000000000000, 0.000000000000000000 ) ) ;
#5820=VECTOR ( 'NONE', #771, 1000.000000000000000 ) ;
#5821=ORIENTED_EDGE ( 'NONE', *, *, #16872, .T. ) ;
#5823=AXIS2_PLACEMENT_3D ( 'NONE', #2732, #14949, #19537 ) ;
#5825=ADVANCED_FACE ( 'NONE', ( #15716 ), #310, .F. ) ;
#5834=ADVANCED_FACE ( 'NONE', ( #3507 ), #3413, .F. ) ;
#5837=DIRECTION ( 'NONE',  ( 1.000000000000000000, 0.000000000000000000, 0.000000000000000000 ) ) ;
#5839=LINE ( 'NONE', #4152, #1307 ) ;
#5842=AXIS2_PLACEMENT_3D ( 'NONE', #14513, #14605, #19094 ) ;
#5848=ORIENTED_EDGE ( 'NONE', *, *, #17371, .T. ) ;
#5858=DIRECTION ( 'NONE',  ( 0.000000000000000000, 0.000000000000000000, -1.000000000000000000 ) ) ;
#5860=CYLINDRICAL_SURFACE ( 'NONE', #12839, 1.000000000000000888 ) ;
#5869=DIRECTION ( 'NONE',  ( 1.000000000000000000, 0.000000000000000000, 0.000000000000000000 ) ) ;
#5870=DIRECTION ( 'NONE',  ( 0.000000000000000000, 0.000000000000000000, -1.000000000000000000 ) ) ;
#5874=LINE ( 'NONE', #2975, #16561 ) ;
#5876=CARTESIAN_POINT ( 'NONE',  ( 5.626241948324195441, -16.73597674598852691, -35.00000000000000000 ) ) ;
#5878=CIRCLE ( 'NONE', #8132, 1.000000000000004441 ) ;
#5879=DIRECTION ( 'NONE',  ( 0.000000000000000000, 0.000000000000000000, 1.000000000000000000 ) ) ;
#5885=DIRECTION ( 'NONE',  ( -0.000000000000000000, -0.000000000000000000, 1.000000000000000000 ) ) ;
#5886=AXIS2_PLACEMENT_3D ( 'NONE', #15313, #7589, #13402 ) ;
#5897=VERTEX_POINT ( 'NONE', #15521 ) ;
#5902=FACE_OUTER_BOUND ( 'NONE', #17006, .T. ) ;
#5909=ORIENTED_EDGE ( 'NONE', *, *, #2004, .T. ) ;
#5920=VECTOR ( 'NONE', #6037, 1000.000000000000000 ) ;
#5929=CYLINDRICAL_SURFACE ( 'NONE', #18614, 1.000000000000002887 ) ;
#5933=CIRCLE ( 'NONE', #14585, 0.9999999999999974465 ) ;
#5945=LINE ( 'NONE', #19454, #3281 ) ;
#5951=CARTESIAN_POINT ( 'NONE',  ( -22.00000000000000355, 0.000000000000000000, -32.00000000000000000 ) ) ;
#5952=VECTOR ( 'NONE', #7677, 1000.000000000000000 ) ;
#5955=ORIENTED_EDGE ( 'NONE', *, *, #74, .T. ) ;
#5957=VERTEX_POINT ( 'NONE', #18907 ) ;
#5960=DIRECTION ( 'NONE',  ( 0.000000000000000000, 0.000000000000000000, 1.000000000000000000 ) ) ;
#5962=CARTESIAN_POINT ( 'NONE',  ( -1.000000000000001998, 18.00000000000000355, 32.00000000000000000 ) ) ;
#5963=CARTESIAN_POINT ( 'NONE',  ( -1.255998204157475318, -17.85806462366060288, -35.00000000000000000 ) ) ;
#5964=ADVANCED_FACE ( 'NONE', ( #518 ), #17419, .F. ) ;
#5966=CARTESIAN_POINT ( 'NONE',  ( 6.626241948324199882, -16.73597674598852691, 35.00000000000000000 ) ) ;
#5967=DIRECTION ( 'NONE',  ( 1.000000000000000000, 0.000000000000000000, 0.000000000000000000 ) ) ;
#5974=CIRCLE ( 'NONE', #5033, 0.9999999999999974465 ) ;
#5981=LINE ( 'NONE', #7274, #7037 ) ;
#5987=CIRCLE ( 'NONE', #13674, 1.000000000000004441 ) ;
#5989=CYLINDRICAL_SURFACE ( 'NONE', #477, 0.9999999999999974465 ) ;
#5991=ORIENTED_EDGE ( 'NONE', *, *, #4030, .F. ) ;
#6004=VERTEX_POINT ( 'NONE', #10020 ) ;
#6006=ADVANCED_FACE ( 'NONE', ( #19011 ), #6982, .F. ) ;
#6018=CARTESIAN_POINT ( 'NONE',  ( 0.000000000000000000, 0.000000000000000000, 29.00000000000000355 ) ) ;
#6037=DIRECTION ( 'NONE',  ( 0.000000000000000000, 0.000000000000000000, -1.000000000000000000 ) ) ;
#6047=CARTESIAN_POINT ( 'NONE',  ( -16.19790265903627713, 9.644882309621941374, 32.00000000000000000 ) ) ;
#6054=CARTESIAN_POINT ( 'NONE',  ( 16.11901729331276556, 5.562305898749055011, 35.00000000000000000 ) ) ;
#6055=EDGE_CURVE ( 'NONE', #8859, #2783, #19104, .T. ) ;
#6061=AXIS2_PLACEMENT_3D ( 'NONE', #4728, #6404, #18435 ) ;
#6062=VERTEX_POINT ( 'NONE', #4195 ) ;
#6070=FACE_BOUND ( 'NONE', #16448, .T. ) ;
#6072=DIRECTION ( 'NONE',  ( 1.000000000000000000, 0.000000000000000000, 0.000000000000000000 ) ) ;
#6074=ORIENTED_EDGE ( 'NONE', *, *, #2158, .T. ) ;
#6082=DIRECTION ( 'NONE',  ( 0.000000000000000000, 0.000000000000000000, 1.000000000000000000 ) ) ;
#6087=CARTESIAN_POINT ( 'NONE',  ( -17.68117051311639898, -3.372863662543042818, -32.00000000000000000 ) ) ;
#6090=DIRECTION ( 'NONE',  ( 0.000000000000000000, 0.000000000000000000, 1.000000000000000000 ) ) ;
#6096=EDGE_LOOP ( 'NONE', ( #5791, #16844, #1405, #1622 ) ) ;
#6097=CYLINDRICAL_SURFACE ( 'NONE', #15080, 12.00000000000000178 ) ;
#6102=EDGE_LOOP ( 'NONE', ( #19557, #3229, #16922, #497 ) ) ;
#6107=CIRCLE ( 'NONE', #9971, 9.000000000000001776 ) ;
#6127=LINE ( 'NONE', #12149, #16072 ) ;
#6132=CARTESIAN_POINT ( 'NONE',  ( 16.19790265903627358, 9.644882309621939598, 32.00000000000000000 ) ) ;
#6135=VECTOR ( 'NONE', #4596, 1000.000000000000000 ) ;
#6141=ORIENTED_EDGE ( 'NONE', *, *, #4599, .F. ) ;
#6144=DIRECTION ( 'NONE',  ( -0.000000000000000000, -0.000000000000000000, 1.000000000000000000 ) ) ;
#6146=EDGE_LOOP ( 'NONE', ( #19663, #330 ) ) ;
#6150=EDGE_CURVE ( 'NONE', #4659, #7585, #16807, .T. ) ;
#6156=AXIS2_PLACEMENT_3D ( 'NONE', #17148, #17343, #9548 ) ;
#6170=CARTESIAN_POINT ( 'NONE',  ( 4.476417968967386862, 17.43449690031536292, 35.00000000000000000 ) ) ;
#6182=CARTESIAN_POINT ( 'NONE',  ( -1.000000000000001998, 18.00000000000000355, -35.00000000000000000 ) ) ;
#6185=CARTESIAN_POINT ( 'NONE',  ( 0.000000000000000000, 0.000000000000000000, 32.00000000000000000 ) ) ;
#6196=CARTESIAN_POINT ( 'NONE',  ( -12.32184790671639085, 13.12143529358541549, 32.00000000000000000 ) ) ;
#6211=EDGE_LOOP ( 'NONE', ( #14715, #7305 ) ) ;
#6215=DIRECTION ( 'NONE',  ( 1.000000000000000000, 0.000000000000000000, 0.000000000000000000 ) ) ;
#6220=DIRECTION ( 'NONE',  ( 0.000000000000000000, 0.000000000000000000, 1.000000000000000000 ) ) ;
#6223=CARTESIAN_POINT ( 'NONE',  ( -13.32184790671639618, 13.12143529358541549, 35.00000000000000000 ) ) ;
#6230=DIRECTION ( 'NONE',  ( 1.000000000000000000, 0.000000000000000000, 0.000000000000000000 ) ) ;
#6238=ORIENTED_EDGE ( 'NONE', *, *, #18421, .T. ) ;
#6241=DIRECTION ( 'NONE',  ( -0.000000000000000000, -0.000000000000000000, 1.000000000000000000 ) ) ;
#6246=DIRECTION ( 'NONE',  ( 1.000000000000000000, 0.000000000000000000, 0.000000000000000000 ) ) ;
#6250=EDGE_CURVE ( 'NONE', #4659, #5172, #7548, .T. ) ;
#6253=LINE ( 'NONE', #18187, #4005 ) ;
#6257=DIRECTION ( 'NONE',  ( 0.000000000000000000, 0.000000000000000000, -1.000000000000000000 ) ) ;
#6261=ORIENTED_EDGE ( 'NONE', *, *, #10207, .T. ) ;
#6264=ADVANCED_FACE ( 'NONE', ( #9590 ), #7873, .F. ) ;
#6268=EDGE_LOOP ( 'NONE', ( #4752, #10576, #6415, #1254 ) ) ;
#6270=EDGE_CURVE ( 'NONE', #2987, #3123, #15882, .T. ) ;
#6285=VECTOR ( 'NONE', #10392, 1000.000000000000000 ) ;
#6290=VERTEX_POINT ( 'NONE', #1690 ) ;
#6292=CARTESIAN_POINT ( 'NONE',  ( 0.000000000000000000, 0.000000000000000000, 35.00000000000000000 ) ) ;
#6299=EDGE_CURVE ( 'NONE', #8343, #4507, #8525, .T. ) ;
#6300=CIRCLE ( 'NONE', #17505, 1.000000000000000888 ) ;
#6304=DIRECTION ( 'NONE',  ( 0.000000000000000000, 0.000000000000000000, -1.000000000000000000 ) ) ;
#6312=DIRECTION ( 'NONE',  ( 0.000000000000000000, 0.000000000000000000, -1.000000000000000000 ) ) ;
#6313=DIRECTION ( 'NONE',  ( 1.000000000000000000, 0.000000000000000000, 0.000000000000000000 ) ) ;
#6324=CARTESIAN_POINT ( 'NONE',  ( 15.19790265903627358, 9.644882309621939598, -32.00000000000000000 ) ) ;
#6343=CARTESIAN_POINT ( 'NONE',  ( -4.476417968967385974, 17.43449690031536292, 32.00000000000000000 ) ) ;
#6346=DIRECTION ( 'NONE',  ( -0.000000000000000000, -0.000000000000000000, 1.000000000000000000 ) ) ;
#6348=FACE_BOUND ( 'NONE', #13390, .T. ) ;
#6352=DIRECTION ( 'NONE',  ( 1.000000000000000000, 0.000000000000000000, 0.000000000000000000 ) ) ;
#6354=ORIENTED_EDGE ( 'NONE', *, *, #11653, .F. ) ;
#6356=DIRECTION ( 'NONE',  ( 0.000000000000000000, 0.000000000000000000, 1.000000000000000000 ) ) ;
#6360=ORIENTED_EDGE ( 'NONE', *, *, #6250, .F. ) ;
#6365=ADVANCED_FACE ( 'NONE', ( #7048 ), #13182, .F. ) ;
#6367=CARTESIAN_POINT ( 'NONE',  ( -9.671566133830877376, 15.77352024078954429, -32.00000000000000000 ) ) ;
#6370=CYLINDRICAL_SURFACE ( 'NONE', #8049, 1.000000000000002665 ) ;
#6380=FACE_OUTER_BOUND ( 'NONE', #9822, .T. ) ;
#6382=DIRECTION ( 'NONE',  ( 1.000000000000000000, 0.000000000000000000, 0.000000000000000000 ) ) ;
#6385=DIRECTION ( 'NONE',  ( 0.000000000000000000, 0.000000000000000000, 1.000000000000000000 ) ) ;
#6386=EDGE_CURVE ( 'NONE', #22, #4121, #970, .T. ) ;
#6388=VERTEX_POINT ( 'NONE', #9898 ) ;
#6393=CARTESIAN_POINT ( 'NONE',  ( 5.510910596163084625E-16, 18.00000000000000355, -32.00000000000000000 ) ) ;
#6395=CIRCLE ( 'NONE', #16006, 12.00000000000000178 ) ;
#6399=EDGE_LOOP ( 'NONE', ( #15961, #6512 ) ) ;
#6400=DIRECTION ( 'NONE',  ( 1.000000000000000000, 0.000000000000000000, 0.000000000000000000 ) ) ;
#6404=DIRECTION ( 'NONE',  ( -0.000000000000000000, -0.000000000000000000, 1.000000000000000000 ) ) ;
#6405=CYLINDRICAL_SURFACE ( 'NONE', #13646, 1.000000000000002665 ) ;
#6406=DIRECTION ( 'NONE',  ( -0.000000000000000000, -0.000000000000000000, 1.000000000000000000 ) ) ;
#6415=ORIENTED_EDGE ( 'NONE', *, *, #4751, .T. ) ;
#6416=CARTESIAN_POINT ( 'NONE',  ( 2.255998204157473097, -17.85806462366060288, -32.00000000000000000 ) ) ;
#6418=EDGE_LOOP ( 'NONE', ( #19219, #18555, #8003, #2047 ) ) ;
#6420=DIRECTION ( 'NONE',  ( -0.000000000000000000, -0.000000000000000000, 1.000000000000000000 ) ) ;
#6421=ORIENTED_EDGE ( 'NONE', *, *, #18205, .T. ) ;
#6428=CARTESIAN_POINT ( 'NONE',  ( -11.32184790671638730, 13.12143529358541549, 35.00000000000000000 ) ) ;
#6429=CARTESIAN_POINT ( 'NONE',  ( 0.000000000000000000, 0.000000000000000000, -30.00000000000000355 ) ) ;
#6434=CARTESIAN_POINT ( 'NONE',  ( -9.580134541264520465, -14.56230589874905235, 35.00000000000000000 ) ) ;
#6437=AXIS2_PLACEMENT_3D ( 'NONE', #12496, #3489, #13900 ) ;
#6438=VERTEX_POINT ( 'NONE', #10480 ) ;
#6442=CIRCLE ( 'NONE', #17325, 0.9999999999999974465 ) ;
#6444=FACE_BOUND ( 'NONE', #13532, .T. ) ;
#6445=EDGE_LOOP ( 'NONE', ( #4164, #10036, #7733, #3220 ) ) ;
#6446=LINE ( 'NONE', #14069, #7555 ) ;
#6447=ORIENTED_EDGE ( 'NONE', *, *, #9297, .T. ) ;
#6452=ADVANCED_FACE ( 'NONE', ( #10383 ), #5860, .F. ) ;
#6456=ORIENTED_EDGE ( 'NONE', *, *, #5135, .T. ) ;
#6459=DIRECTION ( 'NONE',  ( 1.000000000000000000, 0.000000000000000000, 0.000000000000000000 ) ) ;
#6462=DIRECTION ( 'NONE',  ( 0.000000000000000000, 0.000000000000000000, -1.000000000000000000 ) ) ;
#6465=DIRECTION ( 'NONE',  ( -1.000000000000000000, 0.000000000000000000, 0.000000000000000000 ) ) ;
#6476=CARTESIAN_POINT ( 'NONE',  ( 15.28688694438835505, -7.664027248171309203, 32.00000000000000000 ) ) ;
#6481=DIRECTION ( 'NONE',  ( -1.000000000000000000, 0.000000000000000000, -0.000000000000000000 ) ) ;
#6482=ORIENTED_EDGE ( 'NONE', *, *, #17607, .F. ) ;
#6484=CARTESIAN_POINT ( 'NONE',  ( -4.476417968967385974, 17.43449690031536292, 35.00000000000000000 ) ) ;
#6495=LINE ( 'NONE', #15526, #8363 ) ;
#6498=FACE_OUTER_BOUND ( 'NONE', #12928, .T. ) ;
#6501=ORIENTED_EDGE ( 'NONE', *, *, #13356, .F. ) ;
#6502=DIRECTION ( 'NONE',  ( 0.000000000000000000, 0.000000000000000000, -1.000000000000000000 ) ) ;
#6512=ORIENTED_EDGE ( 'NONE', *, *, #5175, .F. ) ;
#6519=AXIS2_PLACEMENT_3D ( 'NONE', #3420, #526, #17324 ) ;
#6521=CYLINDRICAL_SURFACE ( 'NONE', #753, 1.000000000000000888 ) ;
#6533=ORIENTED_EDGE ( 'NONE', *, *, #8183, .F. ) ;
#6535=CARTESIAN_POINT ( 'NONE',  ( 10.58013454126452046, -14.56230589874905412, -32.00000000000000000 ) ) ;
#6546=VERTEX_POINT ( 'NONE', #8642 ) ;
#6552=AXIS2_PLACEMENT_3D ( 'NONE', #2630, #8742, #11841 ) ;
#6558=DIRECTION ( 'NONE',  ( 1.000000000000000000, 0.000000000000000000, 0.000000000000000000 ) ) ;
#6559=DIRECTION ( 'NONE',  ( -1.000000000000000000, 0.000000000000000000, 0.000000000000000000 ) ) ;
#6565=EDGE_CURVE ( 'NONE', #15969, #15613, #2595, .T. ) ;
#6566=CIRCLE ( 'NONE', #7529, 1.000000000000002665 ) ;
#6570=ORIENTED_EDGE ( 'NONE', *, *, #4518, .T. ) ;
#6578=DIRECTION ( 'NONE',  ( 0.000000000000000000, 0.000000000000000000, 1.000000000000000000 ) ) ;
#6582=VECTOR ( 'NONE', #18404, 1000.000000000000000 ) ;
#6583=DIRECTION ( 'NONE',  ( 1.000000000000000000, 0.000000000000000000, 0.000000000000000000 ) ) ;
#6588=DIRECTION ( 'NONE',  ( -1.000000000000000000, 0.000000000000000000, 0.000000000000000000 ) ) ;
#6596=CYLINDRICAL_SURFACE ( 'NONE', #15537, 1.000000000000003553 ) ;
#6599=AXIS2_PLACEMENT_3D ( 'NONE', #7668, #19585, #16894 ) ;
#6605=EDGE_LOOP ( 'NONE', ( #245, #8350 ) ) ;
#6606=FACE_OUTER_BOUND ( 'NONE', #4111, .T. ) ;
#6609=VERTEX_POINT ( 'NONE', #16059 ) ;
#6613=ORIENTED_EDGE ( 'NONE', *, *, #17036, .F. ) ;
#6614=AXIS2_PLACEMENT_3D ( 'NONE', #5191, #16186, #8568 ) ;
#6616=EDGE_CURVE ( 'NONE', #12779, #12621, #16344, .T. ) ;
#6619=EDGE_CURVE ( 'NONE', #14047, #18333, #52, .T. ) ;
#6624=ORIENTED_EDGE ( 'NONE', *, *, #4736, .F. ) ;
#6626=AXIS2_PLACEMENT_3D ( 'NONE', #16592, #10588, #4285 ) ;
#6628=CARTESIAN_POINT ( 'NONE',  ( 1.255998204157470211, -17.85806462366060288, -35.00000000000000000 ) ) ;
#6629=AXIS2_PLACEMENT_3D ( 'NONE', #17630, #11435, #4020 ) ;
#6632=VERTEX_POINT ( 'NONE', #8740 ) ;
#6636=ORIENTED_EDGE ( 'NONE', *, *, #4836, .F. ) ;
#6638=ADVANCED_FACE ( 'NONE', ( #17947 ), #4239, .F. ) ;
#6645=FACE_BOUND ( 'NONE', #17012, .T. ) ;
#6649=FACE_OUTER_BOUND ( 'NONE', #2624, .T. ) ;
#6650=EDGE_CURVE ( 'NONE', #5753, #14722, #11547, .T. ) ;
#6653=DIRECTION ( 'NONE',  ( 1.000000000000000000, 0.000000000000000000, 0.000000000000000000 ) ) ;
#6655=DIRECTION ( 'NONE',  ( 1.000000000000000000, 0.000000000000000000, 0.000000000000000000 ) ) ;
#6656=EDGE_CURVE ( 'NONE', #9320, #13012, #945, .T. ) ;
#6662=ORIENTED_EDGE ( 'NONE', *, *, #17607, .T. ) ;
#6669=CARTESIAN_POINT ( 'NONE',  ( 9.671566133830877376, 15.77352024078954784, -32.00000000000000000 ) ) ;
#6672=CARTESIAN_POINT ( 'NONE',  ( 13.86923836996420789, -11.47363181547641453, -32.00000000000000000 ) ) ;
#6678=LINE ( 'NONE', #9608, #16092 ) ;
#6686=ORIENTED_EDGE ( 'NONE', *, *, #18735, .T. ) ;
#6695=VERTEX_POINT ( 'NONE', #2726 ) ;
#6696=DIRECTION ( 'NONE',  ( -0.000000000000000000, -0.000000000000000000, 1.000000000000000000 ) ) ;
#6703=FACE_OUTER_BOUND ( 'NONE', #2621, .T. ) ;
#6707=CARTESIAN_POINT ( 'NONE',  ( 3.476417968967386418, 17.43449690031536292, 32.00000000000000000 ) ) ;
#6713=FACE_BOUND ( 'NONE', #12167, .T. ) ;
#6714=DIRECTION ( 'NONE',  ( 0.000000000000000000, 0.000000000000000000, -1.000000000000000000 ) ) ;
#6723=ORIENTED_EDGE ( 'NONE', *, *, #17251, .T. ) ;
#6724=DIRECTION ( 'NONE',  ( 1.000000000000000000, 0.000000000000000000, 0.000000000000000000 ) ) ;
#6730=ORIENTED_EDGE ( 'NONE', *, *, #8829, .F. ) ;
#6733=CIRCLE ( 'NONE', #8670, 1.000000000000004441 ) ;
#6736=EDGE_CURVE ( 'NONE', #19457, #19757, #5777, .T. ) ;
#6739=ADVANCED_FACE ( 'NONE', ( #1629 ), #3127, .F. ) ;
#6748=DIRECTION ( 'NONE',  ( 0.000000000000000000, 0.000000000000000000, -1.000000000000000000 ) ) ;
#6753=EDGE_LOOP ( 'NONE', ( #1890, #3304 ) ) ;
#6760=AXIS2_PLACEMENT_3D ( 'NONE', #10867, #3255, #16878 ) ;
#6762=CARTESIAN_POINT ( 'NONE',  ( 0.000000000000000000, 0.000000000000000000, 29.00000000000000355 ) ) ;
#6777=ORIENTED_EDGE ( 'NONE', *, *, #2457, .F. ) ;
#6778=FACE_OUTER_BOUND ( 'NONE', #8867, .T. ) ;
#6779=CARTESIAN_POINT ( 'NONE',  ( -17.96448111170888851, 1.130229351527647585, 35.00000000000000000 ) ) ;
#6799=FILL_AREA_STYLE ('',( #722 ) ) ;
#6807=VERTEX_POINT ( 'NONE', #10445 ) ;
#6810=CARTESIAN_POINT ( 'NONE',  ( 10.58013454126452046, -14.56230589874905412, -32.00000000000000000 ) ) ;
#6812=ORIENTED_EDGE ( 'NONE', *, *, #17088, .T. ) ;
#6814=FACE_BOUND ( 'NONE', #3134, .T. ) ;
#6817=EDGE_CURVE ( 'NONE', #1977, #17754, #6107, .T. ) ;
#6826=EDGE_CURVE ( 'NONE', #9896, #12690, #12044, .T. ) ;
#6832=DIRECTION ( 'NONE',  ( 1.000000000000000000, 0.000000000000000000, 0.000000000000000000 ) ) ;
#6835=ORIENTED_EDGE ( 'NONE', *, *, #4310, .T. ) ;
#6842=ADVANCED_FACE ( 'NONE', ( #3024 ), #14635, .F. ) ;
#6848=CARTESIAN_POINT ( 'NONE',  ( -22.00000000000000355, 0.000000000000000000, -32.00000000000000000 ) ) ;
#6849=AXIS2_PLACEMENT_3D ( 'NONE', #9604, #11000, #18894 ) ;
#6851=ORIENTED_EDGE ( 'NONE', *, *, #7705, .T. ) ;
#6853=ADVANCED_FACE ( 'NONE', ( #16141 ), #7001, .T. ) ;
#6861=EDGE_CURVE ( 'NONE', #6695, #4912, #3726, .T. ) ;
#6862=EDGE_CURVE ( 'NONE', #8877, #3117, #1655, .T. ) ;
#6864=DIRECTION ( 'NONE',  ( 1.000000000000000000, 0.000000000000000000, 0.000000000000000000 ) ) ;
#6874=CARTESIAN_POINT ( 'NONE',  ( 18.11901729331276911, 5.562305898749055011, 32.00000000000000000 ) ) ;
#6884=EDGE_CURVE ( 'NONE', #15039, #9330, #3890, .T. ) ;
#6885=CIRCLE ( 'NONE', #17467, 1.000000000000002665 ) ;
#6887=LINE ( 'NONE', #13017, #7485 ) ;
#6888=EDGE_CURVE ( 'NONE', #17830, #4459, #4533, .T. ) ;
#6891=CARTESIAN_POINT ( 'NONE',  ( 16.11901729331276556, 5.562305898749055011, -32.00000000000000000 ) ) ;
#6904=DIRECTION ( 'NONE',  ( 1.000000000000000000, 0.000000000000000000, 0.000000000000000000 ) ) ;
#6907=DIRECTION ( 'NONE',  ( 1.000000000000000000, 0.000000000000000000, 0.000000000000000000 ) ) ;
#6915=AXIS2_PLACEMENT_3D ( 'NONE', #6018, #8936, #2721 ) ;
#6924=FACE_BOUND ( 'NONE', #17909, .T. ) ;
#6925=EDGE_LOOP ( 'NONE', ( #12040, #18684 ) ) ;
#6930=DIRECTION ( 'NONE',  ( 0.000000000000000000, 0.000000000000000000, 1.000000000000000000 ) ) ;
#6938=EDGE_CURVE ( 'NONE', #4210, #14047, #5222, .T. ) ;
#6940=VERTEX_POINT ( 'NONE', #12935 ) ;
#6945=CARTESIAN_POINT ( 'NONE',  ( 0.000000000000000000, 0.000000000000000000, -35.00000000000000000 ) ) ;
#6951=ORIENTED_EDGE ( 'NONE', *, *, #6938, .F. ) ;
#6956=AXIS2_PLACEMENT_3D ( 'NONE', #19591, #18295, #14897 ) ;
#6959=DIRECTION ( 'NONE',  ( -0.000000000000000000, -0.000000000000000000, 1.000000000000000000 ) ) ;
#6963=FACE_BOUND ( 'NONE', #19273, .T. ) ;
#6967=CIRCLE ( 'NONE', #5687, 1.000000000000003553 ) ;
#6982=CYLINDRICAL_SURFACE ( 'NONE', #19060, 1.000000000000000888 ) ;
#6983=VECTOR ( 'NONE', #4526, 1000.000000000000000 ) ;
#6986=DIRECTION ( 'NONE',  ( 0.000000000000000000, 0.000000000000000000, -1.000000000000000000 ) ) ;
#6990=EDGE_CURVE ( 'NONE', #2257, #3690, #10921, .T. ) ;
#6991=VERTEX_POINT ( 'NONE', #7388 ) ;
#6995=EDGE_LOOP ( 'NONE', ( #2252, #11370, #4868, #3956 ) ) ;
#7001=CYLINDRICAL_SURFACE ( 'NONE', #17622, 22.00000000000000355 ) ;
#7005=FACE_BOUND ( 'NONE', #15215, .T. ) ;
#7014=FACE_OUTER_BOUND ( 'NONE', #11149, .T. ) ;
#7016=DIRECTION ( 'NONE',  ( 0.000000000000000000, 0.000000000000000000, 1.000000000000000000 ) ) ;
#7019=ORIENTED_EDGE ( 'NONE', *, *, #3666, .T. ) ;
#7022=DIRECTION ( 'NONE',  ( 0.000000000000000000, 0.000000000000000000, 1.000000000000000000 ) ) ;
#7024=CARTESIAN_POINT ( 'NONE',  ( -1.255998204157475318, -17.85806462366060288, -32.00000000000000000 ) ) ;
#7029=VECTOR ( 'NONE', #16696, 1000.000000000000000 ) ;
#7037=VECTOR ( 'NONE', #4297, 1000.000000000000000 ) ;
#7038=CARTESIAN_POINT ( 'NONE',  ( 3.255998204157476206, -17.85806462366060288, -35.00000000000000000 ) ) ;
#7040=EDGE_LOOP ( 'NONE', ( #12007, #3745, #8744, #3172 ) ) ;
#7042=DIRECTION ( 'NONE',  ( 0.000000000000000000, 0.000000000000000000, 1.000000000000000000 ) ) ;
#7048=FACE_OUTER_BOUND ( 'NONE', #8160, .T. ) ;
#7050=EDGE_LOOP ( 'NONE', ( #15436, #2878, #2364, #4226 ) ) ;
#7062=EDGE_LOOP ( 'NONE', ( #15932, #17775, #7401, #10162 ) ) ;
#7078=AXIS2_PLACEMENT_3D ( 'NONE', #2270, #15587, #6655 ) ;
#7088=ADVANCED_FACE ( 'NONE', ( #13314 ), #15119, .F. ) ;
#7090=ORIENTED_EDGE ( 'NONE', *, *, #17291, .F. ) ;
#7094=AXIS2_PLACEMENT_3D ( 'NONE', #13975, #13773, #1961 ) ;
#7097=VECTOR ( 'NONE', #11571, 1000.000000000000000 ) ;
#7100=DIRECTION ( 'NONE',  ( 0.000000000000000000, 0.000000000000000000, -1.000000000000000000 ) ) ;
#7101=ORIENTED_EDGE ( 'NONE', *, *, #12099, .F. ) ;
#7108=( GEOMETRIC_REPRESENTATION_CONTEXT ( 3 ) GLOBAL_UNCERTAINTY_ASSIGNED_CONTEXT ( ( #14406 ) ) GLOBAL_UNIT_ASSIGNED_CONTEXT ( ( #17225, #3713, #9737 ) ) REPRESENTATION_CONTEXT ( 'NONE', 'WORKASPACE' ) );
#7121=DIRECTION ( 'NONE',  ( 1.000000000000000000, 0.000000000000000000, 0.000000000000000000 ) ) ;
#7137=AXIS2_PLACEMENT_3D ( 'NONE', #18284, #10682, #19678 ) ;
#7140=ORIENTED_EDGE ( 'NONE', *, *, #12182, .T. ) ;
#7141=LINE ( 'NONE', #5654, #4740 ) ;
#7145=EDGE_LOOP ( 'NONE', ( #6141, #4720 ) ) ;
#7146=FACE_OUTER_BOUND ( 'NONE', #18312, .T. ) ;
#7154=DIRECTION ( 'NONE',  ( 0.000000000000000000, 0.000000000000000000, 1.000000000000000000 ) ) ;
#7157=ADVANCED_FACE ( 'NONE', ( #16723 ), #404, .F. ) ;
#7160=DIRECTION ( 'NONE',  ( 0.000000000000000000, 0.000000000000000000, 1.000000000000000000 ) ) ;
#7172=VERTEX_POINT ( 'NONE', #3406 ) ;
#7174=EDGE_CURVE ( 'NONE', #10470, #10657, #18279, .T. ) ;
#7178=CARTESIAN_POINT ( 'NONE',  ( 18.11901729331276911, 5.562305898749055011, 35.00000000000000000 ) ) ;
#7183=DIRECTION ( 'NONE',  ( 1.000000000000000000, 0.000000000000000000, 0.000000000000000000 ) ) ;
#7189=DIRECTION ( 'NONE',  ( 0.000000000000000000, 0.000000000000000000, 1.000000000000000000 ) ) ;
#7198=ADVANCED_FACE ( 'NONE', ( #1900 ), #6097, .F. ) ;
#7206=CARTESIAN_POINT ( 'NONE',  ( -14.86923836996421144, -11.47363181547641275, 32.00000000000000000 ) ) ;
#7211=CARTESIAN_POINT ( 'NONE',  ( 11.32184790671639263, 13.12143529358541016, 32.00000000000000000 ) ) ;
#7221=EDGE_CURVE ( 'NONE', #2723, #11827, #304, .T. ) ;
#7230=DIRECTION ( 'NONE',  ( 0.000000000000000000, 0.000000000000000000, -1.000000000000000000 ) ) ;
#7231=VECTOR ( 'NONE', #5262, 1000.000000000000000 ) ;
#7235=ORIENTED_EDGE ( 'NONE', *, *, #6650, .T. ) ;
#7237=DIRECTION ( 'NONE',  ( -0.000000000000000000, -0.000000000000000000, 1.000000000000000000 ) ) ;
#7241=EDGE_LOOP ( 'NONE', ( #6624, #2166, #5955, #14014 ) ) ;
#7242=CYLINDRICAL_SURFACE ( 'NONE', #12970, 1.000000000000000888 ) ;
#7244=FACE_OUTER_BOUND ( 'NONE', #1440, .T. ) ;
#7261=CARTESIAN_POINT ( 'NONE',  ( 0.000000000000000000, 0.000000000000000000, 32.00000000000000000 ) ) ;
#7263=EDGE_CURVE ( 'NONE', #10856, #2723, #7381, .T. ) ;
#7271=EDGE_LOOP ( 'NONE', ( #13131, #11769 ) ) ;
#7273=ADVANCED_FACE ( 'NONE', ( #14210 ), #11501, .F. ) ;
#7274=CARTESIAN_POINT ( 'NONE',  ( -13.32184790671639618, 13.12143529358541549, 32.00000000000000000 ) ) ;
#7275=AXIS2_PLACEMENT_3D ( 'NONE', #14771, #1064, #19263 ) ;
#7292=DIRECTION ( 'NONE',  ( -0.000000000000000000, -0.000000000000000000, 1.000000000000000000 ) ) ;
#7304=FACE_BOUND ( 'NONE', #11869, .T. ) ;
#7305=ORIENTED_EDGE ( 'NONE', *, *, #18592, .T. ) ;
#7319=CARTESIAN_POINT ( 'NONE',  ( -5.626241948324210540, -16.73597674598852336, -32.00000000000000000 ) ) ;
#7321=CIRCLE ( 'NONE', #12782, 0.9999999999999974465 ) ;
#7329=ORIENTED_EDGE ( 'NONE', *, *, #7705, .F. ) ;
#7337=EDGE_CURVE ( 'NONE', #10636, #3405, #8052, .T. ) ;
#7341=CIRCLE ( 'NONE', #7999, 1.000000000000000888 ) ;
#7342=ORIENTED_EDGE ( 'NONE', *, *, #7337, .T. ) ;
#7344=VERTEX_POINT ( 'NONE', #11404 ) ;
#7345=CYLINDRICAL_SURFACE ( 'NONE', #8379, 1.000000000000003553 ) ;
#7347=CARTESIAN_POINT ( 'NONE',  ( -17.11901729331276911, 5.562305898749051458, -32.00000000000000000 ) ) ;
#7360=FACE_BOUND ( 'NONE', #5785, .T. ) ;
#7364=CIRCLE ( 'NONE', #16018, 1.000000000000004441 ) ;
#7381=CIRCLE ( 'NONE', #4222, 1.000000000000004441 ) ;
#7383=EDGE_LOOP ( 'NONE', ( #3674, #16892 ) ) ;
#7385=ORIENTED_EDGE ( 'NONE', *, *, #111, .F. ) ;
#7388=CARTESIAN_POINT ( 'NONE',  ( -3.255998204157480203, -17.85806462366060288, -32.00000000000000000 ) ) ;
#7391=DIRECTION ( 'NONE',  ( -0.000000000000000000, -0.000000000000000000, 1.000000000000000000 ) ) ;
#7393=AXIS2_PLACEMENT_3D ( 'NONE', #8515, #10116, #16310 ) ;
#7395=AXIS2_PLACEMENT_3D ( 'NONE', #2959, #3059, #10968 ) ;
#7398=CIRCLE ( 'NONE', #12548, 1.000000000000002665 ) ;
#7401=ORIENTED_EDGE ( 'NONE', *, *, #11166, .T. ) ;
#7412=CIRCLE ( 'NONE', #5823, 1.000000000000002665 ) ;
#7413=DIRECTION ( 'NONE',  ( 0.000000000000000000, 0.000000000000000000, 1.000000000000000000 ) ) ;
#7416=CLOSED_SHELL ( 'NONE', ( #11872, #16151, #15442, #4573, #8849, #1027, #1979, #35, #4639, #7273, #8298, #16705, #42, #19322, #18127, #19345, #5964, #1932, #8432, #14209, #10189, #7607, #19387, #2489, #3531, #5825, #13086, #17674, #16195, #6739, #7157, #14178, #16441, #10720, #12276, #2505, #10483, #15170, #490, #17588, #209, #15926, #17783, #2113, #5401, #4124, #9594, #6006, #6365, #6842, #10145, #12105, #15451, #1952, #1761, #7198, #14608, #4926, #1544, #3382, #6853, #8219, #10323, #12597, #8578, #6638, #5292, #14951, #19227, #18861, #12692, #13936, #3926, #3757, #19617, #7655, #11083, #10281, #19059, #11139, #1276, #9417, #365, #13157, #11292, #8894, #9000, #14784, #18866, #669, #6264, #10737, #3971, #12648, #2440, #5553, #9046, #7088, #2091, #16712, #5168, #8023, #14808, #15707, #18834, #3567, #16556, #17315, #3390, #6452, #15789, #5834, #9514, #16424, #13697, #5379, #18965, #10768 ) ) ;
#7423=ORIENTED_EDGE ( 'NONE', *, *, #13212, .T. ) ;
#7432=CARTESIAN_POINT ( 'NONE',  ( 0.000000000000000000, 0.000000000000000000, 35.00000000000000000 ) ) ;
#7434=DIRECTION ( 'NONE',  ( 1.000000000000000000, 0.000000000000000000, 0.000000000000000000 ) ) ;
#7439=ORIENTED_EDGE ( 'NONE', *, *, #13766, .T. ) ;
#7446=DIRECTION ( 'NONE',  ( 1.000000000000000000, 0.000000000000000000, 0.000000000000000000 ) ) ;
#7475=CARTESIAN_POINT ( 'NONE',  ( -16.19790265903627713, 9.644882309621941374, 32.00000000000000000 ) ) ;
#7478=CARTESIAN_POINT ( 'NONE',  ( -17.28688694438836393, -7.664027248171298545, -32.00000000000000000 ) ) ;
#7479=AXIS2_PLACEMENT_3D ( 'NONE', #11612, #17814, #14530 ) ;
#7485=VECTOR ( 'NONE', #19107, 1000.000000000000000 ) ;
#7486=CARTESIAN_POINT ( 'NONE',  ( 14.19790265903627180, 9.644882309621939598, 32.00000000000000000 ) ) ;
#7491=DIRECTION ( 'NONE',  ( -0.000000000000000000, -0.000000000000000000, 1.000000000000000000 ) ) ;
#7500=CARTESIAN_POINT ( 'NONE',  ( 17.96448111170888851, 1.130229351527639148, -35.00000000000000000 ) ) ;
#7501=CARTESIAN_POINT ( 'NONE',  ( 18.68117051311639543, -3.372863662543048591, -32.00000000000000000 ) ) ;
#7511=ORIENTED_EDGE ( 'NONE', *, *, #4434, .T. ) ;
#7513=VERTEX_POINT ( 'NONE', #4584 ) ;
#7514=DIRECTION ( 'NONE',  ( -0.000000000000000000, -0.000000000000000000, 1.000000000000000000 ) ) ;
#7518=DIRECTION ( 'NONE',  ( 0.000000000000000000, 0.000000000000000000, -1.000000000000000000 ) ) ;
#7522=EDGE_CURVE ( 'NONE', #6004, #10056, #9679, .T. ) ;
#7529=AXIS2_PLACEMENT_3D ( 'NONE', #8720, #10046, #11531 ) ;
#7531=CARTESIAN_POINT ( 'NONE',  ( 16.19790265903627358, 9.644882309621939598, 32.00000000000000000 ) ) ;
#7533=CARTESIAN_POINT ( 'NONE',  ( -11.58013454126452579, -14.56230589874905235, 32.00000000000000000 ) ) ;
#7536=VERTEX_POINT ( 'NONE', #19779 ) ;
#7543=ORIENTED_EDGE ( 'NONE', *, *, #1885, .T. ) ;
#7547=EDGE_CURVE ( 'NONE', #13907, #16740, #4683, .T. ) ;
#7548=CIRCLE ( 'NONE', #5320, 1.000000000000000888 ) ;
#7552=DIRECTION ( 'NONE',  ( -0.000000000000000000, -0.000000000000000000, 1.000000000000000000 ) ) ;
#7555=VECTOR ( 'NONE', #6257, 1000.000000000000000 ) ;
#7558=DIRECTION ( 'NONE',  ( 1.000000000000000000, 0.000000000000000000, 0.000000000000000000 ) ) ;
#7570=EDGE_CURVE ( 'NONE', #13799, #4257, #5184, .T. ) ;
#7575=CIRCLE ( 'NONE', #10158, 1.000000000000004441 ) ;
#7576=EDGE_LOOP ( 'NONE', ( #14764, #7875 ) ) ;
#7579=ORIENTED_EDGE ( 'NONE', *, *, #1143, .T. ) ;
#7585=VERTEX_POINT ( 'NONE', #13986 ) ;
#7589=DIRECTION ( 'NONE',  ( 0.000000000000000000, 0.000000000000000000, 1.000000000000000000 ) ) ;
#7591=( LENGTH_UNIT ( ) NAMED_UNIT ( * ) SI_UNIT ( .MILLI., .METRE. ) );
#7596=EDGE_CURVE ( 'NONE', #18721, #9320, #1990, .T. ) ;
#7598=ORIENTED_EDGE ( 'NONE', *, *, #1019, .T. ) ;
#7604=CARTESIAN_POINT ( 'NONE',  ( 7.626241948324204323, -16.73597674598852691, -32.00000000000000000 ) ) ;
#7606=ORIENTED_EDGE ( 'NONE', *, *, #111, .T. ) ;
#7607=ADVANCED_FACE ( 'NONE', ( #9191 ), #13786, .F. ) ;
#7614=DIRECTION ( 'NONE',  ( 0.000000000000000000, 0.000000000000000000, 1.000000000000000000 ) ) ;
#7617=ORIENTED_EDGE ( 'NONE', *, *, #13847, .T. ) ;
#7627=VERTEX_POINT ( 'NONE', #3276 ) ;
#7628=DIRECTION ( 'NONE',  ( -0.000000000000000000, -0.000000000000000000, 1.000000000000000000 ) ) ;
#7633=VERTEX_POINT ( 'NONE', #9392 ) ;
#7635=CARTESIAN_POINT ( 'NONE',  ( 15.28688694438835505, -7.664027248171309203, -35.00000000000000000 ) ) ;
#7636=ORIENTED_EDGE ( 'NONE', *, *, #7174, .T. ) ;
#7640=SURFACE_STYLE_USAGE ( .BOTH. , #15361 ) ;
#7642=LINE ( 'NONE', #13757, #12611 ) ;
#7647=ORIENTED_EDGE ( 'NONE', *, *, #4310, .F. ) ;
#7653=CARTESIAN_POINT ( 'NONE',  ( -1.000000000000001998, 18.00000000000000355, 32.00000000000000000 ) ) ;
#7654=VERTEX_POINT ( 'NONE', #3178 ) ;
#7655=ADVANCED_FACE ( 'NONE', ( #9288 ), #15391, .F. ) ;
#7657=CARTESIAN_POINT ( 'NONE',  ( -9.671566133830877376, 15.77352024078954429, -32.00000000000000000 ) ) ;
#7659=ORIENTED_EDGE ( 'NONE', *, *, #4982, .T. ) ;
#7665=DIRECTION ( 'NONE',  ( 1.000000000000000000, 0.000000000000000000, 0.000000000000000000 ) ) ;
#7668=CARTESIAN_POINT ( 'NONE',  ( 0.000000000000000000, 0.000000000000000000, -35.00000000000000000 ) ) ;
#7670=CARTESIAN_POINT ( 'NONE',  ( 0.000000000000000000, 0.000000000000000000, 29.00000000000000355 ) ) ;
#7677=DIRECTION ( 'NONE',  ( 0.000000000000000000, 0.000000000000000000, -1.000000000000000000 ) ) ;
#7683=EDGE_CURVE ( 'NONE', #12225, #8623, #19548, .T. ) ;
#7691=VERTEX_POINT ( 'NONE', #15886 ) ;
#7694=CARTESIAN_POINT ( 'NONE',  ( -16.11901729331276911, 5.562305898749051458, -35.00000000000000000 ) ) ;
#7696=CARTESIAN_POINT ( 'NONE',  ( -13.32184790671639618, 13.12143529358541549, -35.00000000000000000 ) ) ;
#7700=EDGE_LOOP ( 'NONE', ( #12235, #15731 ) ) ;
#7705=EDGE_CURVE ( 'NONE', #9739, #12760, #7742, .T. ) ;
#7712=ORIENTED_EDGE ( 'NONE', *, *, #7953, .T. ) ;
#7715=EDGE_LOOP ( 'NONE', ( #8147, #15727 ) ) ;
#7718=FACE_OUTER_BOUND ( 'NONE', #11351, .T. ) ;
#7720=FACE_OUTER_BOUND ( 'NONE', #4817, .T. ) ;
#7724=CIRCLE ( 'NONE', #389, 1.000000000000003553 ) ;
#7726=VERTEX_POINT ( 'NONE', #11081 ) ;
#7727=AXIS2_PLACEMENT_3D ( 'NONE', #2507, #4313, #1310 ) ;
#7733=ORIENTED_EDGE ( 'NONE', *, *, #16716, .F. ) ;
#7735=DIRECTION ( 'NONE',  ( 0.000000000000000000, 0.000000000000000000, 1.000000000000000000 ) ) ;
#7742=CIRCLE ( 'NONE', #7078, 1.000000000000000888 ) ;
#7743=( NAMED_UNIT ( * ) PLANE_ANGLE_UNIT ( ) SI_UNIT ( $, .RADIAN. ) );
#7756=ORIENTED_EDGE ( 'NONE', *, *, #13377, .F. ) ;
#7765=DIRECTION ( 'NONE',  ( 0.000000000000000000, 0.000000000000000000, 1.000000000000000000 ) ) ;
#7766=ORIENTED_EDGE ( 'NONE', *, *, #9565, .T. ) ;
#7770=DIRECTION ( 'NONE',  ( 0.000000000000000000, 0.000000000000000000, 1.000000000000000000 ) ) ;
#7772=VERTEX_POINT ( 'NONE', #12587 ) ;
#7776=CIRCLE ( 'NONE', #18964, 1.000000000000003553 ) ;
#7777=CARTESIAN_POINT ( 'NONE',  ( -2.255998204157477538, -17.85806462366060288, 32.00000000000000000 ) ) ;
#7780=ORIENTED_EDGE ( 'NONE', *, *, #2356, .T. ) ;
#7786=EDGE_CURVE ( 'NONE', #3138, #17485, #13151, .T. ) ;
#7794=ORIENTED_EDGE ( 'NONE', *, *, #12939, .F. ) ;
#7800=EDGE_LOOP ( 'NONE', ( #18272, #7636 ) ) ;
#7805=AXIS2_PLACEMENT_3D ( 'NONE', #6185, #16820, #12311 ) ;
#7811=LINE ( 'NONE', #18815, #3242 ) ;
#7814=DIRECTION ( 'NONE',  ( 1.000000000000000000, 0.000000000000000000, 0.000000000000000000 ) ) ;
#7817=EDGE_LOOP ( 'NONE', ( #16531, #11155 ) ) ;
#7819=DIRECTION ( 'NONE',  ( -1.000000000000000000, 0.000000000000000000, 0.000000000000000000 ) ) ;
#7820=ORIENTED_EDGE ( 'NONE', *, *, #4736, .T. ) ;
#7822=CARTESIAN_POINT ( 'NONE',  ( -4.476417968967385974, 17.43449690031536292, -35.00000000000000000 ) ) ;
#7823=ORIENTED_EDGE ( 'NONE', *, *, #8558, .F. ) ;
#7825=CYLINDRICAL_SURFACE ( 'NONE', #16856, 1.000000000000003553 ) ;
#7826=AXIS2_PLACEMENT_3D ( 'NONE', #10287, #2760, #8577 ) ;
#7831=ORIENTED_EDGE ( 'NONE', *, *, #11409, .F. ) ;
#7861=CARTESIAN_POINT ( 'NONE',  ( 3.255998204157476206, -17.85806462366060288, -32.00000000000000000 ) ) ;
#7872=DIRECTION ( 'NONE',  ( -0.000000000000000000, -0.000000000000000000, 1.000000000000000000 ) ) ;
#7873=CYLINDRICAL_SURFACE ( 'NONE', #16841, 1.000000000000000888 ) ;
#7875=ORIENTED_EDGE ( 'NONE', *, *, #17394, .F. ) ;
#7876=CARTESIAN_POINT ( 'NONE',  ( -17.68117051311639898, -3.372863662543042818, 32.00000000000000000 ) ) ;
#7878=EDGE_CURVE ( 'NONE', #8143, #12225, #1541, .T. ) ;
#7891=VECTOR ( 'NONE', #6748, 1000.000000000000000 ) ;
#7898=DIRECTION ( 'NONE',  ( 0.000000000000000000, 0.000000000000000000, -1.000000000000000000 ) ) ;
#7899=ORIENTED_EDGE ( 'NONE', *, *, #3515, .T. ) ;
#7905=AXIS2_PLACEMENT_3D ( 'NONE', #10522, #16618, #2900 ) ;
#7907=DIRECTION ( 'NONE',  ( 0.000000000000000000, 0.000000000000000000, 1.000000000000000000 ) ) ;
#7911=EDGE_CURVE ( 'NONE', #5740, #13049, #6127, .T. ) ;
#7919=CARTESIAN_POINT ( 'NONE',  ( 0.000000000000000000, 0.000000000000000000, 32.00000000000000000 ) ) ;
#7923=CIRCLE ( 'NONE', #15605, 22.00000000000000355 ) ;
#7926=DIRECTION ( 'NONE',  ( 1.000000000000000000, 0.000000000000000000, 0.000000000000000000 ) ) ;
#7933=ORIENTED_EDGE ( 'NONE', *, *, #18788, .T. ) ;
#7936=EDGE_CURVE ( 'NONE', #7585, #9689, #8992, .T. ) ;
#7945=ORIENTED_EDGE ( 'NONE', *, *, #127, .T. ) ;
#7948=EDGE_LOOP ( 'NONE', ( #4368, #8565, #12594, #6482 ) ) ;
#7953=EDGE_CURVE ( 'NONE', #19421, #19054, #13644, .T. ) ;
#7954=CARTESIAN_POINT ( 'NONE',  ( 15.19790265903627358, 9.644882309621939598, -32.00000000000000000 ) ) ;
#7955=FACE_BOUND ( 'NONE', #12888, .T. ) ;
#7969=EDGE_CURVE ( 'NONE', #18235, #10647, #7412, .T. ) ;
#7975=EDGE_LOOP ( 'NONE', ( #14028, #18041 ) ) ;
#7981=FACE_OUTER_BOUND ( 'NONE', #3484, .T. ) ;
#7984=ORIENTED_EDGE ( 'NONE', *, *, #13484, .T. ) ;
#7995=ORIENTED_EDGE ( 'NONE', *, *, #19101, .F. ) ;
#7999=AXIS2_PLACEMENT_3D ( 'NONE', #18600, #18311, #1704 ) ;
#8003=ORIENTED_EDGE ( 'NONE', *, *, #3554, .T. ) ;
#8005=CARTESIAN_POINT ( 'NONE',  ( 5.510910596163084625E-16, 18.00000000000000355, -32.00000000000000000 ) ) ;
#8007=CIRCLE ( 'NONE', #5758, 9.000000000000000000 ) ;
#8008=CARTESIAN_POINT ( 'NONE',  ( -16.11901729331276911, 5.562305898749051458, 32.00000000000000000 ) ) ;
#8023=ADVANCED_FACE ( 'NONE', ( #13543 ), #5929, .F. ) ;
#8024=AXIS2_PLACEMENT_3D ( 'NONE', #11940, #7413, #6215 ) ;
#8025=LINE ( 'NONE', #742, #9041 ) ;
#8033=ORIENTED_EDGE ( 'NONE', *, *, #4637, .T. ) ;
#8035=CIRCLE ( 'NONE', #4529, 1.000000000000003109 ) ;
#8041=ORIENTED_EDGE ( 'NONE', *, *, #13088, .F. ) ;
#8043=DIRECTION ( 'NONE',  ( -0.000000000000000000, -0.000000000000000000, 1.000000000000000000 ) ) ;
#8044=CARTESIAN_POINT ( 'NONE',  ( -12.86923836996420611, -11.47363181547641275, -32.00000000000000000 ) ) ;
#8049=AXIS2_PLACEMENT_3D ( 'NONE', #8186, #5080, #11193 ) ;
#8051=CIRCLE ( 'NONE', #5495, 1.000000000000002442 ) ;
#8052=CIRCLE ( 'NONE', #9356, 1.000000000000002665 ) ;
#8055=AXIS2_PLACEMENT_3D ( 'NONE', #9464, #18652, #15559 ) ;
#8057=FACE_BOUND ( 'NONE', #18921, .T. ) ;
#8068=VECTOR ( 'NONE', #6220, 1000.000000000000000 ) ;
#8071=AXIS2_PLACEMENT_3D ( 'NONE', #6324, #14343, #12553 ) ;
#8074=CARTESIAN_POINT ( 'NONE',  ( 16.28688694438835327, -7.664027248171309203, -32.00000000000000000 ) ) ;
#8078=EDGE_LOOP ( 'NONE', ( #15182, #13856 ) ) ;
#8079=DIRECTION ( 'NONE',  ( 1.000000000000000000, 0.000000000000000000, 0.000000000000000000 ) ) ;
#8081=CARTESIAN_POINT ( 'NONE',  ( -13.32184790671639618, 13.12143529358541549, 32.00000000000000000 ) ) ;
#8083=CARTESIAN_POINT ( 'NONE',  ( -16.28688694438836038, -7.664027248171298545, -35.00000000000000000 ) ) ;
#8088=CIRCLE ( 'NONE', #10648, 1.000000000000000888 ) ;
#8090=ORIENTED_EDGE ( 'NONE', *, *, #13212, .F. ) ;
#8092=CARTESIAN_POINT ( 'NONE',  ( 15.28688694438835505, -7.664027248171309203, 32.00000000000000000 ) ) ;
#8109=EDGE_CURVE ( 'NONE', #10470, #3148, #9447, .T. ) ;
#8115=CARTESIAN_POINT ( 'NONE',  ( 16.19790265903627358, 9.644882309621939598, 35.00000000000000000 ) ) ;
#8117=ORIENTED_EDGE ( 'NONE', *, *, #5643, .T. ) ;
#8127=DIRECTION ( 'NONE',  ( 1.000000000000000000, 0.000000000000000000, 0.000000000000000000 ) ) ;
#8128=DIRECTION ( 'NONE',  ( 0.000000000000000000, 0.000000000000000000, -1.000000000000000000 ) ) ;
#8129=ORIENTED_EDGE ( 'NONE', *, *, #1955, .T. ) ;
#8131=CARTESIAN_POINT ( 'NONE',  ( 16.28688694438835327, -7.664027248171309203, 32.00000000000000000 ) ) ;
#8132=AXIS2_PLACEMENT_3D ( 'NONE', #14351, #17647, #8544 ) ;
#8134=DIRECTION ( 'NONE',  ( 1.000000000000000000, 0.000000000000000000, 0.000000000000000000 ) ) ;
#8143=VERTEX_POINT ( 'NONE', #3434 ) ;
#8146=CIRCLE ( 'NONE', #10706, 1.000000000000000888 ) ;
#8147=ORIENTED_EDGE ( 'NONE', *, *, #13095, .F. ) ;
#8159=CIRCLE ( 'NONE', #13903, 1.000000000000004441 ) ;
#8160=EDGE_LOOP ( 'NONE', ( #2637, #18948, #468, #16573 ) ) ;
#8161=CIRCLE ( 'NONE', #11672, 1.000000000000004441 ) ;
#8164=FACE_BOUND ( 'NONE', #5742, .T. ) ;
#8165=EDGE_LOOP ( 'NONE', ( #12609, #5224 ) ) ;
#8174=AXIS2_PLACEMENT_3D ( 'NONE', #3773, #584, #967 ) ;
#8182=EDGE_CURVE ( 'NONE', #13666, #16380, #412, .T. ) ;
#8183=EDGE_CURVE ( 'NONE', #15108, #12385, #11590, .T. ) ;
#8185=AXIS2_PLACEMENT_3D ( 'NONE', #5516, #13319, #19420 ) ;
#8186=CARTESIAN_POINT ( 'NONE',  ( -10.58013454126452224, -14.56230589874905235, -32.00000000000000000 ) ) ;
#8187=CARTESIAN_POINT ( 'NONE',  ( -8.671566133830875600, 15.77352024078954429, -32.00000000000000000 ) ) ;
#8195=DIRECTION ( 'NONE',  ( 1.000000000000000000, 0.000000000000000000, 0.000000000000000000 ) ) ;
#8197=PRODUCT_DEFINITION_CONTEXT ( 'detailed design', #13155, 'design' ) ;
#8198=DIRECTION ( 'NONE',  ( 1.000000000000000000, 0.000000000000000000, 0.000000000000000000 ) ) ;
#8203=AXIS2_PLACEMENT_3D ( 'NONE', #11907, #2593, #1202 ) ;
#8204=CARTESIAN_POINT ( 'NONE',  ( 1.000000000000003331, 18.00000000000000355, 32.00000000000000000 ) ) ;
#8205=ORIENTED_EDGE ( 'NONE', *, *, #11604, .F. ) ;
#8208=EDGE_LOOP ( 'NONE', ( #14307, #6238 ) ) ;
#8214=CIRCLE ( 'NONE', #15891, 1.000000000000003109 ) ;
#8218=CIRCLE ( 'NONE', #4061, 1.000000000000003109 ) ;
#8219=ADVANCED_FACE ( 'NONE', ( #2127, #3628, #837, #738, #1014, #17730, #12740, #5419, #15841, #8231, #17339, #636, #7005, #6814, #5325, #8530, #13129, #9750, #8329, #6713, #13035, #4023, #19220, #11528, #14439, #19035, #12835 ), #18933, .F. ) ;
#8221=CARTESIAN_POINT ( 'NONE',  ( -12.00000000000000178, 0.000000000000000000, 29.00000000000000355 ) ) ;
#8222=ORIENTED_EDGE ( 'NONE', *, *, #13174, .F. ) ;
#8224=DIRECTION ( 'NONE',  ( 1.000000000000000000, 0.000000000000000000, 0.000000000000000000 ) ) ;
#8228=CARTESIAN_POINT ( 'NONE',  ( 7.671566133830872047, 15.77352024078954784, 32.00000000000000000 ) ) ;
#8230=EDGE_LOOP ( 'NONE', ( #18111, #15419, #666, #14770 ) ) ;
#8231=FACE_BOUND ( 'NONE', #10018, .T. ) ;
#8240=ORIENTED_EDGE ( 'NONE', *, *, #14921, .F. ) ;
#8245=CARTESIAN_POINT ( 'NONE',  ( -12.32184790671639085, 13.12143529358541549, -35.00000000000000000 ) ) ;
#8247=ORIENTED_EDGE ( 'NONE', *, *, #13583, .F. ) ;
#8253=EDGE_LOOP ( 'NONE', ( #18383, #5821, #8985, #5405 ) ) ;
#8262=EDGE_LOOP ( 'NONE', ( #8476, #11822 ) ) ;
#8278=CARTESIAN_POINT ( 'NONE',  ( -8.671566133830875600, 15.77352024078954429, 32.00000000000000000 ) ) ;
#8279=DIRECTION ( 'NONE',  ( 0.000000000000000000, 0.000000000000000000, 1.000000000000000000 ) ) ;
#8281=CARTESIAN_POINT ( 'NONE',  ( 18.96448111170889206, 1.130229351527639148, 35.00000000000000000 ) ) ;
#8285=DIRECTION ( 'NONE',  ( 0.000000000000000000, 0.000000000000000000, 1.000000000000000000 ) ) ;
#8286=DIRECTION ( 'NONE',  ( 0.000000000000000000, 0.000000000000000000, 1.000000000000000000 ) ) ;
#8293=ORIENTED_EDGE ( 'NONE', *, *, #15204, .F. ) ;
#8298=ADVANCED_FACE ( 'NONE', ( #10334 ), #13318, .F. ) ;
#8307=CYLINDRICAL_SURFACE ( 'NONE', #17090, 1.000000000000002665 ) ;
#8308=AXIS2_PLACEMENT_3D ( 'NONE', #4331, #16542, #5817 ) ;
#8309=EDGE_CURVE ( 'NONE', #4750, #5566, #17317, .T. ) ;
#8310=CARTESIAN_POINT ( 'NONE',  ( 0.000000000000000000, 0.000000000000000000, 29.00000000000000355 ) ) ;
#8316=EDGE_LOOP ( 'NONE', ( #5315, #586, #7766, #15534 ) ) ;
#8324=DIRECTION ( 'NONE',  ( 0.000000000000000000, 0.000000000000000000, 1.000000000000000000 ) ) ;
#8327=CARTESIAN_POINT ( 'NONE',  ( -6.626241948324210540, -16.73597674598852336, -32.00000000000000000 ) ) ;
#8328=ORIENTED_EDGE ( 'NONE', *, *, #10326, .F. ) ;
#8329=FACE_BOUND ( 'NONE', #13929, .T. ) ;
#8336=DIRECTION ( 'NONE',  ( 0.000000000000000000, 0.000000000000000000, -1.000000000000000000 ) ) ;
#8343=VERTEX_POINT ( 'NONE', #4910 ) ;
#8346=ORIENTED_EDGE ( 'NONE', *, *, #19101, .T. ) ;
#8350=ORIENTED_EDGE ( 'NONE', *, *, #5422, .T. ) ;
#8359=AXIS2_PLACEMENT_3D ( 'NONE', #14749, #2246, #7121 ) ;
#8363=VECTOR ( 'NONE', #1812, 1000.000000000000000 ) ;
#8371=DIRECTION ( 'NONE',  ( 0.000000000000000000, 0.000000000000000000, 1.000000000000000000 ) ) ;
#8372=ORIENTED_EDGE ( 'NONE', *, *, #8183, .T. ) ;
#8379=AXIS2_PLACEMENT_3D ( 'NONE', #8774, #13080, #5463 ) ;
#8393=CARTESIAN_POINT ( 'NONE',  ( -18.68117051311639543, -3.372863662543042818, -32.00000000000000000 ) ) ;
#8395=VECTOR ( 'NONE', #8848, 1000.000000000000000 ) ;
#8402=DIRECTION ( 'NONE',  ( -0.000000000000000000, -0.000000000000000000, 1.000000000000000000 ) ) ;
#8415=DIRECTION ( 'NONE',  ( 0.000000000000000000, 0.000000000000000000, 1.000000000000000000 ) ) ;
#8424=ORIENTED_EDGE ( 'NONE', *, *, #13948, .F. ) ;
#8425=FACE_OUTER_BOUND ( 'NONE', #4734, .T. ) ;
#8431=CYLINDRICAL_SURFACE ( 'NONE', #9924, 1.000000000000004441 ) ;
#8432=ADVANCED_FACE ( 'NONE', ( #3799 ), #17606, .F. ) ;
#8435=CARTESIAN_POINT ( 'NONE',  ( 0.000000000000000000, 0.000000000000000000, 32.00000000000000000 ) ) ;
#8438=VERTEX_POINT ( 'NONE', #3998 ) ;
#8439=DIRECTION ( 'NONE',  ( 1.000000000000000000, 0.000000000000000000, 0.000000000000000000 ) ) ;
#8443=DIRECTION ( 'NONE',  ( 0.000000000000000000, 0.000000000000000000, 1.000000000000000000 ) ) ;
#8450=FACE_BOUND ( 'NONE', #8612, .T. ) ;
#8452=EDGE_LOOP ( 'NONE', ( #9073, #19432 ) ) ;
#8458=CARTESIAN_POINT ( 'NONE',  ( -15.19790265903627180, 9.644882309621941374, -35.00000000000000000 ) ) ;
#8459=ORIENTED_EDGE ( 'NONE', *, *, #9588, .T. ) ;
#8462=AXIS2_PLACEMENT_3D ( 'NONE', #14556, #14652, #3743 ) ;
#8464=ORIENTED_EDGE ( 'NONE', *, *, #14468, .F. ) ;
#8476=ORIENTED_EDGE ( 'NONE', *, *, #2287, .F. ) ;
#8478=EDGE_CURVE ( 'NONE', #5711, #18074, #17636, .T. ) ;
#8480=CARTESIAN_POINT ( 'NONE',  ( 5.626241948324195441, -16.73597674598852691, 32.00000000000000000 ) ) ;
#8481=CIRCLE ( 'NONE', #19653, 1.000000000000000888 ) ;
#8493=DIRECTION ( 'NONE',  ( 1.000000000000000000, 0.000000000000000000, 0.000000000000000000 ) ) ;
#8506=EDGE_LOOP ( 'NONE', ( #11164, #5333, #2890, #764 ) ) ;
#8514=CARTESIAN_POINT ( 'NONE',  ( -14.19790265903626647, 9.644882309621941374, -32.00000000000000000 ) ) ;
#8515=CARTESIAN_POINT ( 'NONE',  ( 4.476417968967386862, 17.43449690031536292, 32.00000000000000000 ) ) ;
#8516=DIRECTION ( 'NONE',  ( 1.000000000000000000, 0.000000000000000000, 0.000000000000000000 ) ) ;
#8525=CIRCLE ( 'NONE', #18428, 12.00000000000000178 ) ;
#8528=CARTESIAN_POINT ( 'NONE',  ( -8.671566133830875600, 15.77352024078954429, -32.00000000000000000 ) ) ;
#8529=VERTEX_POINT ( 'NONE', #10205 ) ;
#8530=FACE_BOUND ( 'NONE', #10911, .T. ) ;
#8535=CIRCLE ( 'NONE', #10773, 1.000000000000000888 ) ;
#8538=ORIENTED_EDGE ( 'NONE', *, *, #1149, .T. ) ;
#8542=FACE_BOUND ( 'NONE', #1966, .T. ) ;
#8543=ORIENTED_EDGE ( 'NONE', *, *, #12633, .F. ) ;
#8544=DIRECTION ( 'NONE',  ( 1.000000000000000000, 0.000000000000000000, 0.000000000000000000 ) ) ;
#8554=AXIS2_PLACEMENT_3D ( 'NONE', #5249, #12964, #3653 ) ;
#8557=ORIENTED_EDGE ( 'NONE', *, *, #14677, .T. ) ;
#8558=EDGE_CURVE ( 'NONE', #13272, #4315, #10501, .T. ) ;
#8560=AXIS2_PLACEMENT_3D ( 'NONE', #8528, #10332, #14636 ) ;
#8565=ORIENTED_EDGE ( 'NONE', *, *, #13701, .T. ) ;
#8568=DIRECTION ( 'NONE',  ( -1.000000000000000000, 0.000000000000000000, 0.000000000000000000 ) ) ;
#8569=EDGE_CURVE ( 'NONE', #10979, #19457, #16600, .T. ) ;
#8576=VERTEX_POINT ( 'NONE', #4292 ) ;
#8577=DIRECTION ( 'NONE',  ( 1.000000000000000000, 0.000000000000000000, 0.000000000000000000 ) ) ;
#8578=ADVANCED_FACE ( 'NONE', ( #8896 ), #13294, .F. ) ;
#8579=DIRECTION ( 'NONE',  ( 0.000000000000000000, 0.000000000000000000, 1.000000000000000000 ) ) ;
#8582=CIRCLE ( 'NONE', #16587, 22.00000000000000355 ) ;
#8598=DIRECTION ( 'NONE',  ( -0.000000000000000000, -0.000000000000000000, 1.000000000000000000 ) ) ;
#8602=CARTESIAN_POINT ( 'NONE',  ( -14.19790265903626647, 9.644882309621941374, 32.00000000000000000 ) ) ;
#8607=EDGE_LOOP ( 'NONE', ( #1289, #17108 ) ) ;
#8608=CARTESIAN_POINT ( 'NONE',  ( -6.626241948324210540, -16.73597674598852336, 35.00000000000000000 ) ) ;
#8612=EDGE_LOOP ( 'NONE', ( #916, #19524 ) ) ;
#8613=CARTESIAN_POINT ( 'NONE',  ( 10.58013454126452046, -14.56230589874905412, 32.00000000000000000 ) ) ;
#8619=CARTESIAN_POINT ( 'NONE',  ( 11.58013454126452579, -14.56230589874905412, -35.00000000000000000 ) ) ;
#8623=VERTEX_POINT ( 'NONE', #10890 ) ;
#8633=FACE_BOUND ( 'NONE', #2917, .T. ) ;
#8634=EDGE_CURVE ( 'NONE', #4629, #5305, #5480, .T. ) ;
#8635=ORIENTED_EDGE ( 'NONE', *, *, #10886, .F. ) ;
#8637=ORIENTED_EDGE ( 'NONE', *, *, #6299, .F. ) ;
#8642=CARTESIAN_POINT ( 'NONE',  ( 16.96448111170888851, 1.130229351527639370, 32.00000000000000000 ) ) ;
#8650=DIRECTION ( 'NONE',  ( 0.000000000000000000, 0.000000000000000000, 1.000000000000000000 ) ) ;
#8665=ORIENTED_EDGE ( 'NONE', *, *, #6055, .T. ) ;
#8670=AXIS2_PLACEMENT_3D ( 'NONE', #5126, #2034, #17054 ) ;
#8671=ORIENTED_EDGE ( 'NONE', *, *, #5422, .F. ) ;
#8673=VECTOR ( 'NONE', #19292, 1000.000000000000000 ) ;
#8676=CARTESIAN_POINT ( 'NONE',  ( -5.626241948324210540, -16.73597674598852336, -35.00000000000000000 ) ) ;
#8680=CARTESIAN_POINT ( 'NONE',  ( -7.671566133830872047, 15.77352024078954429, 35.00000000000000000 ) ) ;
#8683=ORIENTED_EDGE ( 'NONE', *, *, #16066, .T. ) ;
#8693=EDGE_LOOP ( 'NONE', ( #7090, #10374, #3699, #7423 ) ) ;
#8695=VECTOR ( 'NONE', #982, 1000.000000000000000 ) ;
#8699=DIRECTION ( 'NONE',  ( 1.000000000000000000, 0.000000000000000000, 0.000000000000000000 ) ) ;
#8700=AXIS2_PLACEMENT_3D ( 'NONE', #12993, #8579, #11393 ) ;
#8708=DIRECTION ( 'NONE',  ( -1.000000000000000000, 0.000000000000000000, 0.000000000000000000 ) ) ;
#8709=EDGE_LOOP ( 'NONE', ( #10336, #16094 ) ) ;
#8716=VECTOR ( 'NONE', #18766, 1000.000000000000000 ) ;
#8720=CARTESIAN_POINT ( 'NONE',  ( 5.510910596163084625E-16, 18.00000000000000355, 35.00000000000000000 ) ) ;
#8725=CARTESIAN_POINT ( 'NONE',  ( 4.476417968967386862, 17.43449690031536292, 32.00000000000000000 ) ) ;
#8733=LINE ( 'NONE', #7206, #8752 ) ;
#8734=ORIENTED_EDGE ( 'NONE', *, *, #19165, .T. ) ;
#8740=CARTESIAN_POINT ( 'NONE',  ( -3.476417968967383754, 17.43449690031536292, 32.00000000000000000 ) ) ;
#8742=DIRECTION ( 'NONE',  ( 0.000000000000000000, 0.000000000000000000, -1.000000000000000000 ) ) ;
#8744=ORIENTED_EDGE ( 'NONE', *, *, #4850, .F. ) ;
#8747=DIRECTION ( 'NONE',  ( 0.000000000000000000, 0.000000000000000000, 1.000000000000000000 ) ) ;
#8748=EDGE_CURVE ( 'NONE', #3405, #10636, #5166, .T. ) ;
#8752=VECTOR ( 'NONE', #13329, 1000.000000000000000 ) ;
#8757=EDGE_CURVE ( 'NONE', #16011, #15888, #7724, .T. ) ;
#8759=ORIENTED_EDGE ( 'NONE', *, *, #84, .T. ) ;
#8762=CIRCLE ( 'NONE', #19302, 1.000000000000002442 ) ;
#8765=DIRECTION ( 'NONE',  ( 0.000000000000000000, 0.000000000000000000, 1.000000000000000000 ) ) ;
#8768=DIRECTION ( 'NONE',  ( -1.000000000000000000, 0.000000000000000000, 0.000000000000000000 ) ) ;
#8771=ORIENTED_EDGE ( 'NONE', *, *, #8829, .T. ) ;
#8773=VERTEX_POINT ( 'NONE', #17583 ) ;
#8774=CARTESIAN_POINT ( 'NONE',  ( -8.671566133830875600, 15.77352024078954429, 32.00000000000000000 ) ) ;
#8779=EDGE_CURVE ( 'NONE', #14268, #3988, #10298, .T. ) ;
#8780=CIRCLE ( 'NONE', #160, 0.9999999999999974465 ) ;
#8799=VERTEX_POINT ( 'NONE', #4979 ) ;
#8804=CIRCLE ( 'NONE', #834, 1.000000000000004441 ) ;
#8807=ORIENTED_EDGE ( 'NONE', *, *, #17366, .T. ) ;
#8817=AXIS2_PLACEMENT_3D ( 'NONE', #17964, #2939, #14957 ) ;
#8822=EDGE_CURVE ( 'NONE', #17152, #8438, #2303, .T. ) ;
#8823=PRODUCT_DEFINITION ( 'UNKNOWN', '', #5071, #8197 ) ;
#8826=EDGE_CURVE ( 'NONE', #17528, #17855, #18596, .T. ) ;
#8829=EDGE_CURVE ( 'NONE', #10056, #6004, #14776, .T. ) ;
#8831=VECTOR ( 'NONE', #9832, 1000.000000000000000 ) ;
#8835=AXIS2_PLACEMENT_3D ( 'NONE', #11115, #18516, #6588 ) ;
#8840=ORIENTED_EDGE ( 'NONE', *, *, #2897, .T. ) ;
#8847=ORIENTED_EDGE ( 'NONE', *, *, #2197, .F. ) ;
#8848=DIRECTION ( 'NONE',  ( 0.000000000000000000, 0.000000000000000000, 1.000000000000000000 ) ) ;
#8849=ADVANCED_FACE ( 'NONE', ( #5660 ), #2558, .F. ) ;
#8851=EDGE_CURVE ( 'NONE', #17102, #2419, #8051, .T. ) ;
#8857=DIRECTION ( 'NONE',  ( 0.000000000000000000, 0.000000000000000000, 1.000000000000000000 ) ) ;
#8859=VERTEX_POINT ( 'NONE', #16377 ) ;
#8867=EDGE_LOOP ( 'NONE', ( #13414, #16218, #17420, #6447 ) ) ;
#8869=DIRECTION ( 'NONE',  ( 1.000000000000000000, 0.000000000000000000, 0.000000000000000000 ) ) ;
#8870=CYLINDRICAL_SURFACE ( 'NONE', #6614, 1.000000000000004441 ) ;
#8873=ORIENTED_EDGE ( 'NONE', *, *, #15833, .T. ) ;
#8877=VERTEX_POINT ( 'NONE', #13368 ) ;
#8886=EDGE_LOOP ( 'NONE', ( #8543, #10861, #4909, #5614 ) ) ;
#8889=FACE_BOUND ( 'NONE', #17563, .T. ) ;
#8894=ADVANCED_FACE ( 'NONE', ( #7244 ), #7345, .F. ) ;
#8896=FACE_OUTER_BOUND ( 'NONE', #4854, .T. ) ;
#8902=CARTESIAN_POINT ( 'NONE',  ( 9.671566133830877376, 15.77352024078954784, 32.00000000000000000 ) ) ;
#8904=EDGE_LOOP ( 'NONE', ( #15073, #12913, #4012, #6851 ) ) ;
#8909=DIRECTION ( 'NONE',  ( 1.000000000000000000, 0.000000000000000000, 0.000000000000000000 ) ) ;
#8913=CARTESIAN_POINT ( 'NONE',  ( 15.28688694438835505, -7.664027248171309203, -32.00000000000000000 ) ) ;
#8927=VERTEX_POINT ( 'NONE', #15074 ) ;
#8936=DIRECTION ( 'NONE',  ( 0.000000000000000000, 0.000000000000000000, 1.000000000000000000 ) ) ;
#8937=ORIENTED_EDGE ( 'NONE', *, *, #2557, .T. ) ;
#8943=EDGE_CURVE ( 'NONE', #3123, #2987, #4221, .T. ) ;
#8951=DIRECTION ( 'NONE',  ( 1.000000000000000000, 0.000000000000000000, 0.000000000000000000 ) ) ;
#8956=EDGE_LOOP ( 'NONE', ( #971, #10661 ) ) ;
#8960=EDGE_CURVE ( 'NONE', #600, #15138, #4270, .T. ) ;
#8964=DIRECTION ( 'NONE',  ( -0.000000000000000000, -0.000000000000000000, 1.000000000000000000 ) ) ;
#8966=CARTESIAN_POINT ( 'NONE',  ( -18.68117051311639543, -3.372863662543042818, 32.00000000000000000 ) ) ;
#8973=ORIENTED_EDGE ( 'NONE', *, *, #8822, .F. ) ;
#8974=EDGE_CURVE ( 'NONE', #4210, #5957, #9676, .T. ) ;
#8980=ORIENTED_EDGE ( 'NONE', *, *, #4030, .T. ) ;
#8981=LINE ( 'NONE', #15086, #17147 ) ;
#8983=EDGE_CURVE ( 'NONE', #11811, #16968, #17008, .T. ) ;
#8985=ORIENTED_EDGE ( 'NONE', *, *, #14235, .T. ) ;
#8986=DIRECTION ( 'NONE',  ( 0.000000000000000000, 0.000000000000000000, -1.000000000000000000 ) ) ;
#8987=FACE_BOUND ( 'NONE', #16703, .T. ) ;
#8992=CIRCLE ( 'NONE', #1958, 1.000000000000000888 ) ;
#8995=AXIS2_PLACEMENT_3D ( 'NONE', #14562, #6930, #5439 ) ;
#9000=ADVANCED_FACE ( 'NONE', ( #18466 ), #9074, .F. ) ;
#9002=CARTESIAN_POINT ( 'NONE',  ( -11.32184790671638730, 13.12143529358541549, -32.00000000000000000 ) ) ;
#9003=DIRECTION ( 'NONE',  ( 1.000000000000000000, 0.000000000000000000, 0.000000000000000000 ) ) ;
#9004=EDGE_LOOP ( 'NONE', ( #9026, #16691 ) ) ;
#9009=CYLINDRICAL_SURFACE ( 'NONE', #10879, 1.000000000000005995 ) ;
#9011=CARTESIAN_POINT ( 'NONE',  ( 5.626241948324195441, -16.73597674598852691, 35.00000000000000000 ) ) ;
#9015=EDGE_CURVE ( 'NONE', #11304, #13799, #12076, .T. ) ;
#9021=EDGE_LOOP ( 'NONE', ( #16987, #8033, #2619, #15310 ) ) ;
#9022=AXIS2_PLACEMENT_3D ( 'NONE', #18883, #11287, #15686 ) ;
#9023=AXIS2_PLACEMENT_3D ( 'NONE', #12606, #3687, #17401 ) ;
#9026=ORIENTED_EDGE ( 'NONE', *, *, #17752, .T. ) ;
#9030=EDGE_CURVE ( 'NONE', #10900, #3614, #1987, .T. ) ;
#9031=ORIENTED_EDGE ( 'NONE', *, *, #3106, .F. ) ;
#9041=VECTOR ( 'NONE', #19039, 1000.000000000000000 ) ;
#9046=ADVANCED_FACE ( 'NONE', ( #18275 ), #18564, .F. ) ;
#9048=EDGE_CURVE ( 'NONE', #14720, #4121, #3903, .T. ) ;
#9055=DIRECTION ( 'NONE',  ( -1.000000000000000000, 0.000000000000000000, 0.000000000000000000 ) ) ;
#9058=CARTESIAN_POINT ( 'NONE',  ( 9.000000000000000000, 0.000000000000000000, 35.00000000000000000 ) ) ;
#9063=DIRECTION ( 'NONE',  ( 0.000000000000000000, 0.000000000000000000, 1.000000000000000000 ) ) ;
#9067=DIRECTION ( 'NONE',  ( 0.000000000000000000, 0.000000000000000000, 1.000000000000000000 ) ) ;
#9073=ORIENTED_EDGE ( 'NONE', *, *, #1840, .F. ) ;
#9074=CYLINDRICAL_SURFACE ( 'NONE', #12541, 1.000000000000002665 ) ;
#9079=AXIS2_PLACEMENT_3D ( 'NONE', #4572, #16884, #3165 ) ;
#9089=ORIENTED_EDGE ( 'NONE', *, *, #16757, .T. ) ;
#9090=DIRECTION ( 'NONE',  ( -0.000000000000000000, -0.000000000000000000, -1.000000000000000000 ) ) ;
#9092=CARTESIAN_POINT ( 'NONE',  ( 1.255998204157470211, -17.85806462366060288, -32.00000000000000000 ) ) ;
#9094=DIRECTION ( 'NONE',  ( 1.000000000000000000, 0.000000000000000000, 0.000000000000000000 ) ) ;
#9100=EDGE_CURVE ( 'NONE', #4315, #15354, #4237, .T. ) ;
#9101=ORIENTED_EDGE ( 'NONE', *, *, #18788, .F. ) ;
#9104=CIRCLE ( 'NONE', #5886, 1.000000000000004441 ) ;
#9106=CARTESIAN_POINT ( 'NONE',  ( 5.510910596163084625E-16, 18.00000000000000355, 32.00000000000000000 ) ) ;
#9108=VERTEX_POINT ( 'NONE', #6054 ) ;
#9109=AXIS2_PLACEMENT_3D ( 'NONE', #2488, #16121, #17611 ) ;
#9110=LINE ( 'NONE', #4450, #2064 ) ;
#9115=CYLINDRICAL_SURFACE ( 'NONE', #18225, 1.000000000000004441 ) ;
#9119=CARTESIAN_POINT ( 'NONE',  ( -9.580134541264520465, -14.56230589874905235, -32.00000000000000000 ) ) ;
#9123=VECTOR ( 'NONE', #16381, 1000.000000000000000 ) ;
#9125=CIRCLE ( 'NONE', #2998, 1.000000000000002665 ) ;
#9136=CIRCLE ( 'NONE', #14887, 1.000000000000000888 ) ;
#9167=AXIS2_PLACEMENT_3D ( 'NONE', #2283, #11492, #499 ) ;
#9171=CARTESIAN_POINT ( 'NONE',  ( -12.32184790671639085, 13.12143529358541549, 32.00000000000000000 ) ) ;
#9189=FACE_OUTER_BOUND ( 'NONE', #4064, .T. ) ;
#9191=FACE_OUTER_BOUND ( 'NONE', #18260, .T. ) ;
#9194=CARTESIAN_POINT ( 'NONE',  ( 16.11901729331276556, 5.562305898749055011, 32.00000000000000000 ) ) ;
#9201=ORIENTED_EDGE ( 'NONE', *, *, #1500, .F. ) ;
#9209=DIRECTION ( 'NONE',  ( 0.000000000000000000, 0.000000000000000000, 1.000000000000000000 ) ) ;
#9211=CIRCLE ( 'NONE', #4733, 1.000000000000000888 ) ;
#9214=LINE ( 'NONE', #3196, #15447 ) ;
#9215=EDGE_CURVE ( 'NONE', #3690, #15613, #14950, .T. ) ;
#9219=DIRECTION ( 'NONE',  ( 0.000000000000000000, 0.000000000000000000, 1.000000000000000000 ) ) ;
#9221=ORIENTED_EDGE ( 'NONE', *, *, #13135, .F. ) ;
#9224=CIRCLE ( 'NONE', #9541, 0.9999999999999974465 ) ;
#9225=EDGE_LOOP ( 'NONE', ( #16785, #3609, #15227, #19185 ) ) ;
#9231=FACE_OUTER_BOUND ( 'NONE', #14442, .T. ) ;
#9236=AXIS2_PLACEMENT_3D ( 'NONE', #4435, #27, #1999 ) ;
#9238=ORIENTED_EDGE ( 'NONE', *, *, #11112, .T. ) ;
#9246=VECTOR ( 'NONE', #17410, 1000.000000000000000 ) ;
#9262=DIRECTION ( 'NONE',  ( 0.000000000000000000, 0.000000000000000000, 1.000000000000000000 ) ) ;
#9265=EDGE_LOOP ( 'NONE', ( #5775, #10136, #4830, #19291 ) ) ;
#9266=CARTESIAN_POINT ( 'NONE',  ( 6.626241948324199882, -16.73597674598852691, -35.00000000000000000 ) ) ;
#9270=EDGE_CURVE ( 'NONE', #7513, #1540, #15819, .T. ) ;
#9273=LINE ( 'NONE', #3857, #5820 ) ;
#9280=AXIS2_PLACEMENT_3D ( 'NONE', #15800, #2382, #505 ) ;
#9287=CARTESIAN_POINT ( 'NONE',  ( -3.255998204157480203, -17.85806462366060288, -35.00000000000000000 ) ) ;
#9288=FACE_OUTER_BOUND ( 'NONE', #4532, .T. ) ;
#9292=DIRECTION ( 'NONE',  ( 1.000000000000000000, 0.000000000000000000, 0.000000000000000000 ) ) ;
#9297=EDGE_CURVE ( 'NONE', #8927, #11311, #8146, .T. ) ;
#9300=LINE ( 'NONE', #195, #1720 ) ;
#9301=EDGE_CURVE ( 'NONE', #16271, #16569, #10074, .T. ) ;
#9302=ORIENTED_EDGE ( 'NONE', *, *, #6565, .T. ) ;
#9306=SURFACE_SIDE_STYLE ('',( #297 ) ) ;
#9308=CARTESIAN_POINT ( 'NONE',  ( 7.671566133830872047, 15.77352024078954784, -32.00000000000000000 ) ) ;
#9312=VECTOR ( 'NONE', #19242, 1000.000000000000000 ) ;
#9313=CARTESIAN_POINT ( 'NONE',  ( 1.255998204157470211, -17.85806462366060288, -32.00000000000000000 ) ) ;
#9319=CARTESIAN_POINT ( 'NONE',  ( -5.476417968967388639, 17.43449690031536292, -32.00000000000000000 ) ) ;
#9320=VERTEX_POINT ( 'NONE', #11751 ) ;
#9326=EDGE_LOOP ( 'NONE', ( #5680, #953, #983, #1757 ) ) ;
#9328=LINE ( 'NONE', #12135, #10362 ) ;
#9330=VERTEX_POINT ( 'NONE', #15148 ) ;
#9338=CARTESIAN_POINT ( 'NONE',  ( -1.255998204157475318, -17.85806462366060288, 35.00000000000000000 ) ) ;
#9339=DIRECTION ( 'NONE',  ( 0.000000000000000000, 0.000000000000000000, 1.000000000000000000 ) ) ;
#9350=CARTESIAN_POINT ( 'NONE',  ( 11.58013454126452579, -14.56230589874905412, -32.00000000000000000 ) ) ;
#9352=ORIENTED_EDGE ( 'NONE', *, *, #744, .T. ) ;
#9356=AXIS2_PLACEMENT_3D ( 'NONE', #6484, #2293, #11109 ) ;
#9364=ORIENTED_EDGE ( 'NONE', *, *, #10069, .T. ) ;
#9371=COLOUR_RGB ( '', 0.72549020, 0.75294118, 0.79215686) ;
#9375=CIRCLE ( 'NONE', #8071, 1.000000000000000888 ) ;
#9380=FACE_BOUND ( 'NONE', #7145, .T. ) ;
#9386=VERTEX_POINT ( 'NONE', #10547 ) ;
#9392=CARTESIAN_POINT ( 'NONE',  ( -5.626241948324210540, -16.73597674598852336, 35.00000000000000000 ) ) ;
#9405=DIRECTION ( 'NONE',  ( 1.000000000000000000, 0.000000000000000000, 0.000000000000000000 ) ) ;
#9410=LINE ( 'NONE', #12313, #2255 ) ;
#9411=ORIENTED_EDGE ( 'NONE', *, *, #17001, .F. ) ;
#9416=DIRECTION ( 'NONE',  ( 0.000000000000000000, 0.000000000000000000, 1.000000000000000000 ) ) ;
#9417=ADVANCED_FACE ( 'NONE', ( #18443 ), #10844, .F. ) ;
#9422=AXIS2_PLACEMENT_3D ( 'NONE', #17031, #5015, #5105 ) ;
#9429=CARTESIAN_POINT ( 'NONE',  ( -16.68117051311640253, -3.372863662543042818, -35.00000000000000000 ) ) ;
#9432=ORIENTED_EDGE ( 'NONE', *, *, #8960, .F. ) ;
#9436=CARTESIAN_POINT ( 'NONE',  ( -7.626241948324210540, -16.73597674598852336, 35.00000000000000000 ) ) ;
#9439=EDGE_LOOP ( 'NONE', ( #9547, #11152 ) ) ;
#9440=DIRECTION ( 'NONE',  ( 1.000000000000000000, 0.000000000000000000, 0.000000000000000000 ) ) ;
#9447=LINE ( 'NONE', #16853, #8068 ) ;
#9464=CARTESIAN_POINT ( 'NONE',  ( 5.510910596163084625E-16, 18.00000000000000355, -35.00000000000000000 ) ) ;
#9475=DIRECTION ( 'NONE',  ( 0.000000000000000000, 0.000000000000000000, 1.000000000000000000 ) ) ;
#9479=FACE_BOUND ( 'NONE', #19756, .T. ) ;
#9481=EDGE_LOOP ( 'NONE', ( #672, #18412 ) ) ;
#9482=CARTESIAN_POINT ( 'NONE',  ( -3.476417968967383754, 17.43449690031536292, 32.00000000000000000 ) ) ;
#9501=FACE_OUTER_BOUND ( 'NONE', #17986, .T. ) ;
#9509=SURFACE_STYLE_USAGE ( .BOTH. , #9306 ) ;
#9513=CARTESIAN_POINT ( 'NONE',  ( -18.96448111170889206, 1.130229351527647585, -32.00000000000000000 ) ) ;
#9514=ADVANCED_FACE ( 'NONE', ( #17421 ), #8307, .F. ) ;
#9516=CARTESIAN_POINT ( 'NONE',  ( 15.19790265903627358, 9.644882309621939598, 32.00000000000000000 ) ) ;
#9518=ORIENTED_EDGE ( 'NONE', *, *, #10121, .F. ) ;
#9521=VERTEX_POINT ( 'NONE', #17050 ) ;
#9523=DIRECTION ( 'NONE',  ( -1.000000000000000000, 0.000000000000000000, 0.000000000000000000 ) ) ;
#9526=CIRCLE ( 'NONE', #7905, 0.9999999999999974465 ) ;
#9532=ORIENTED_EDGE ( 'NONE', *, *, #6990, .F. ) ;
#9533=FACE_OUTER_BOUND ( 'NONE', #2454, .T. ) ;
#9534=EDGE_LOOP ( 'NONE', ( #11041, #7820, #5111, #16230 ) ) ;
#9539=FACE_OUTER_BOUND ( 'NONE', #1770, .T. ) ;
#9540=CARTESIAN_POINT ( 'NONE',  ( -17.96448111170888851, 1.130229351527647585, 32.00000000000000000 ) ) ;
#9541=AXIS2_PLACEMENT_3D ( 'NONE', #2749, #16574, #14968 ) ;
#9547=ORIENTED_EDGE ( 'NONE', *, *, #13135, .T. ) ;
#9548=DIRECTION ( 'NONE',  ( 1.000000000000000000, 0.000000000000000000, 0.000000000000000000 ) ) ;
#9552=EDGE_CURVE ( 'NONE', #15782, #19176, #6887, .T. ) ;
#9558=EDGE_CURVE ( 'NONE', #14379, #12547, #14218, .T. ) ;
#9559=VERTEX_POINT ( 'NONE', #8602 ) ;
#9562=DIRECTION ( 'NONE',  ( -1.000000000000000000, 0.000000000000000000, 0.000000000000000000 ) ) ;
#9565=EDGE_CURVE ( 'NONE', #4459, #7726, #2396, .T. ) ;
#9573=EDGE_CURVE ( 'NONE', #15108, #5313, #17904, .T. ) ;
#9576=FACE_BOUND ( 'NONE', #17488, .T. ) ;
#9577=ORIENTED_EDGE ( 'NONE', *, *, #7263, .F. ) ;
#9588=EDGE_CURVE ( 'NONE', #3997, #13012, #8159, .T. ) ;
#9590=FACE_OUTER_BOUND ( 'NONE', #15607, .T. ) ;
#9591=ORIENTED_EDGE ( 'NONE', *, *, #5000, .T. ) ;
#9594=ADVANCED_FACE ( 'NONE', ( #18103 ), #16306, .F. ) ;
#9595=CIRCLE ( 'NONE', #10229, 1.000000000000000888 ) ;
#9598=AXIS2_PLACEMENT_3D ( 'NONE', #319, #12631, #6400 ) ;
#9602=VERTEX_POINT ( 'NONE', #12494 ) ;
#9604=CARTESIAN_POINT ( 'NONE',  ( 17.11901729331276556, 5.562305898749055011, -35.00000000000000000 ) ) ;
#9608=CARTESIAN_POINT ( 'NONE',  ( -5.626241948324210540, -16.73597674598852336, 32.00000000000000000 ) ) ;
#9615=LINE ( 'NONE', #12809, #585 ) ;
#9628=AXIS2_PLACEMENT_3D ( 'NONE', #4694, #17098, #4891 ) ;
#9639=CYLINDRICAL_SURFACE ( 'NONE', #13104, 1.000000000000002665 ) ;
#9640=CARTESIAN_POINT ( 'NONE',  ( -16.68117051311640253, -3.372863662543042818, -32.00000000000000000 ) ) ;
#9641=CARTESIAN_POINT ( 'NONE',  ( -16.19790265903627713, 9.644882309621941374, -32.00000000000000000 ) ) ;
#9645=CYLINDRICAL_SURFACE ( 'NONE', #16814, 9.000000000000001776 ) ;
#9646=AXIS2_PLACEMENT_3D ( 'NONE', #16356, #2638, #2738 ) ;
#9648=AXIS2_PLACEMENT_3D ( 'NONE', #18679, #4976, #17184 ) ;
#9649=VECTOR ( 'NONE', #17437, 1000.000000000000000 ) ;
#9652=DIRECTION ( 'NONE',  ( -1.000000000000000000, 0.000000000000000000, 0.000000000000000000 ) ) ;
#9653=DIRECTION ( 'NONE',  ( 0.000000000000000000, 0.000000000000000000, 1.000000000000000000 ) ) ;
#9659=CIRCLE ( 'NONE', #61, 1.000000000000004441 ) ;
#9666=VERTEX_POINT ( 'NONE', #4888 ) ;
#9668=CARTESIAN_POINT ( 'NONE',  ( 7.626241948324204323, -16.73597674598852691, 32.00000000000000000 ) ) ;
#9669=EDGE_CURVE ( 'NONE', #3614, #10900, #19015, .T. ) ;
#9671=AXIS2_PLACEMENT_3D ( 'NONE', #13581, #5870, #17994 ) ;
#9676=CIRCLE ( 'NONE', #15738, 1.000000000000004441 ) ;
#9679=CIRCLE ( 'NONE', #17338, 9.000000000000000000 ) ;
#9680=CYLINDRICAL_SURFACE ( 'NONE', #9902, 0.9999999999999974465 ) ;
#9687=CARTESIAN_POINT ( 'NONE',  ( -16.96448111170888851, 1.130229351527647808, -32.00000000000000000 ) ) ;
#9689=VERTEX_POINT ( 'NONE', #13696 ) ;
#9697=DIRECTION ( 'NONE',  ( 1.000000000000000000, 0.000000000000000000, 0.000000000000000000 ) ) ;
#9699=DIRECTION ( 'NONE',  ( 0.000000000000000000, 0.000000000000000000, -1.000000000000000000 ) ) ;
#9705=STYLED_ITEM ( 'NONE', ( #12725 ), #12355 ) ;
#9706=CARTESIAN_POINT ( 'NONE',  ( 0.000000000000000000, 0.000000000000000000, -32.00000000000000000 ) ) ;
#9707=DIRECTION ( 'NONE',  ( 1.000000000000000000, 0.000000000000000000, 0.000000000000000000 ) ) ;
#9710=DIRECTION ( 'NONE',  ( 1.000000000000000000, 0.000000000000000000, 0.000000000000000000 ) ) ;
#9722=EDGE_CURVE ( 'NONE', #7172, #16673, #16095, .T. ) ;
#9726=ORIENTED_EDGE ( 'NONE', *, *, #13709, .F. ) ;
#9728=DIRECTION ( 'NONE',  ( 0.000000000000000000, 0.000000000000000000, -1.000000000000000000 ) ) ;
#9729=VERTEX_POINT ( 'NONE', #19177 ) ;
#9737=( NAMED_UNIT ( * ) SI_UNIT ( $, .STERADIAN. ) SOLID_ANGLE_UNIT ( ) );
#9739=VERTEX_POINT ( 'NONE', #8281 ) ;
#9741=ORIENTED_EDGE ( 'NONE', *, *, #3012, .F. ) ;
#9744=DIRECTION ( 'NONE',  ( -1.000000000000000000, 0.000000000000000000, 0.000000000000000000 ) ) ;
#9746=DIRECTION ( 'NONE',  ( 0.000000000000000000, 0.000000000000000000, -1.000000000000000000 ) ) ;
#9749=ORIENTED_EDGE ( 'NONE', *, *, #19676, .F. ) ;
#9750=FACE_BOUND ( 'NONE', #9439, .T. ) ;
#9752=CIRCLE ( 'NONE', #1108, 1.000000000000000888 ) ;
#9753=ORIENTED_EDGE ( 'NONE', *, *, #5643, .F. ) ;
#9755=CARTESIAN_POINT ( 'NONE',  ( -17.96448111170888851, 1.130229351527647585, -32.00000000000000000 ) ) ;
#9756=AXIS2_PLACEMENT_3D ( 'NONE', #6672, #12798, #295 ) ;
#9780=ORIENTED_EDGE ( 'NONE', *, *, #17071, .T. ) ;
#9782=CARTESIAN_POINT ( 'NONE',  ( 10.58013454126452046, -14.56230589874905412, -35.00000000000000000 ) ) ;
#9785=CARTESIAN_POINT ( 'NONE',  ( -5.476417968967388639, 17.43449690031536292, -35.00000000000000000 ) ) ;
#9801=DIRECTION ( 'NONE',  ( 0.000000000000000000, 0.000000000000000000, -1.000000000000000000 ) ) ;
#9802=AXIS2_PLACEMENT_3D ( 'NONE', #524, #10826, #3118 ) ;
#9805=FACE_OUTER_BOUND ( 'NONE', #14948, .T. ) ;
#9812=EDGE_CURVE ( 'NONE', #9108, #18640, #8481, .T. ) ;
#9819=AXIS2_PLACEMENT_3D ( 'NONE', #17496, #10098, #9710 ) ;
#9821=AXIS2_PLACEMENT_3D ( 'NONE', #1776, #6356, #15489 ) ;
#9822=EDGE_LOOP ( 'NONE', ( #14839, #8205, #9238, #4291 ) ) ;
#9824=DIRECTION ( 'NONE',  ( 1.000000000000000000, 0.000000000000000000, 0.000000000000000000 ) ) ;
#9832=DIRECTION ( 'NONE',  ( 0.000000000000000000, 0.000000000000000000, 1.000000000000000000 ) ) ;
#9833=DIRECTION ( 'NONE',  ( 0.000000000000000000, 0.000000000000000000, 1.000000000000000000 ) ) ;
#9852=CIRCLE ( 'NONE', #13341, 1.000000000000004441 ) ;
#9856=DIRECTION ( 'NONE',  ( 0.000000000000000000, 0.000000000000000000, -1.000000000000000000 ) ) ;
#9857=DIRECTION ( 'NONE',  ( 0.000000000000000000, 0.000000000000000000, 1.000000000000000000 ) ) ;
#9858=CARTESIAN_POINT ( 'NONE',  ( -17.11901729331276911, 5.562305898749051458, 32.00000000000000000 ) ) ;
#9861=LINE ( 'NONE', #15951, #19655 ) ;
#9864=ORIENTED_EDGE ( 'NONE', *, *, #13001, .T. ) ;
#9879=EDGE_CURVE ( 'NONE', #3823, #11476, #16158, .T. ) ;
#9880=AXIS2_PLACEMENT_3D ( 'NONE', #18072, #8964, #10472 ) ;
#9882=DIRECTION ( 'NONE',  ( 0.000000000000000000, 0.000000000000000000, -1.000000000000000000 ) ) ;
#9884=CARTESIAN_POINT ( 'NONE',  ( 18.11901729331276911, 5.562305898749055011, -32.00000000000000000 ) ) ;
#9896=VERTEX_POINT ( 'NONE', #17782 ) ;
#9897=DIRECTION ( 'NONE',  ( 0.000000000000000000, 0.000000000000000000, 1.000000000000000000 ) ) ;
#9898=CARTESIAN_POINT ( 'NONE',  ( -16.11901729331276911, 5.562305898749051458, 35.00000000000000000 ) ) ;
#9902=AXIS2_PLACEMENT_3D ( 'NONE', #10075, #17859, #11656 ) ;
#9904=FACE_OUTER_BOUND ( 'NONE', #14091, .T. ) ;
#9905=CARTESIAN_POINT ( 'NONE',  ( 15.28688694438835505, -7.664027248171309203, 35.00000000000000000 ) ) ;
#9924=AXIS2_PLACEMENT_3D ( 'NONE', #829, #3915, #16227 ) ;
#9936=CARTESIAN_POINT ( 'NONE',  ( -6.626241948324210540, -16.73597674598852336, -32.00000000000000000 ) ) ;
#9939=ORIENTED_EDGE ( 'NONE', *, *, #3212, .T. ) ;
#9941=COLOUR_RGB ( '', 0.72549020, 0.75294118, 0.79215686) ;
#9956=DIRECTION ( 'NONE',  ( 0.000000000000000000, 0.000000000000000000, -1.000000000000000000 ) ) ;
#9965=ORIENTED_EDGE ( 'NONE', *, *, #10073, .F. ) ;
#9970=VERTEX_POINT ( 'NONE', #1076 ) ;
#9971=AXIS2_PLACEMENT_3D ( 'NONE', #16547, #15042, #13537 ) ;
#9981=EDGE_CURVE ( 'NONE', #6991, #17102, #13279, .T. ) ;
#9988=DIRECTION ( 'NONE',  ( 1.000000000000000000, 0.000000000000000000, 0.000000000000000000 ) ) ;
#10000=CARTESIAN_POINT ( 'NONE',  ( -12.32184790671639085, 13.12143529358541549, 32.00000000000000000 ) ) ;
#10006=EDGE_CURVE ( 'NONE', #4548, #11655, #498, .T. ) ;
#10013=CARTESIAN_POINT ( 'NONE',  ( 16.96448111170888851, 1.130229351527639370, 32.00000000000000000 ) ) ;
#10018=EDGE_LOOP ( 'NONE', ( #355, #10850 ) ) ;
#10020=CARTESIAN_POINT ( 'NONE',  ( -9.000000000000000000, 1.102182119232617714E-15, 29.00000000000000355 ) ) ;
#10029=DIRECTION ( 'NONE',  ( 0.000000000000000000, 0.000000000000000000, 1.000000000000000000 ) ) ;
#10031=DIRECTION ( 'NONE',  ( 1.000000000000000000, 0.000000000000000000, 0.000000000000000000 ) ) ;
#10032=CARTESIAN_POINT ( 'NONE',  ( 1.255998204157470211, -17.85806462366060288, 35.00000000000000000 ) ) ;
#10036=ORIENTED_EDGE ( 'NONE', *, *, #18513, .T. ) ;
#10037=DIRECTION ( 'NONE',  ( 1.000000000000000000, 0.000000000000000000, 0.000000000000000000 ) ) ;
#10041=FACE_OUTER_BOUND ( 'NONE', #7948, .T. ) ;
#10043=ORIENTED_EDGE ( 'NONE', *, *, #8943, .T. ) ;
#10046=DIRECTION ( 'NONE',  ( 0.000000000000000000, 0.000000000000000000, 1.000000000000000000 ) ) ;
#10053=DIRECTION ( 'NONE',  ( -0.000000000000000000, -0.000000000000000000, 1.000000000000000000 ) ) ;
#10054=FACE_BOUND ( 'NONE', #3833, .T. ) ;
#10056=VERTEX_POINT ( 'NONE', #17751 ) ;
#10058=DIRECTION ( 'NONE',  ( 1.000000000000000000, 0.000000000000000000, 0.000000000000000000 ) ) ;
#10064=DIRECTION ( 'NONE',  ( -0.000000000000000000, -0.000000000000000000, 1.000000000000000000 ) ) ;
#10066=AXIS2_PLACEMENT_3D ( 'NONE', #10269, #3962, #12973 ) ;
#10068=VERTEX_POINT ( 'NONE', #11551 ) ;
#10069=EDGE_CURVE ( 'NONE', #16569, #3939, #3948, .T. ) ;
#10071=CIRCLE ( 'NONE', #12288, 9.000000000000000000 ) ;
#10073=EDGE_CURVE ( 'NONE', #3037, #18092, #18399, .T. ) ;
#10074=CIRCLE ( 'NONE', #3990, 1.000000000000004441 ) ;
#10075=CARTESIAN_POINT ( 'NONE',  ( 13.86923836996420789, -11.47363181547641453, 32.00000000000000000 ) ) ;
#10098=DIRECTION ( 'NONE',  ( -0.000000000000000000, -0.000000000000000000, 1.000000000000000000 ) ) ;
#10103=DIRECTION ( 'NONE',  ( -0.000000000000000000, -0.000000000000000000, 1.000000000000000000 ) ) ;
#10109=CARTESIAN_POINT ( 'NONE',  ( -11.32184790671638730, 13.12143529358541549, 32.00000000000000000 ) ) ;
#10116=DIRECTION ( 'NONE',  ( 0.000000000000000000, 0.000000000000000000, 1.000000000000000000 ) ) ;
#10121=EDGE_CURVE ( 'NONE', #9330, #15039, #19347, .T. ) ;
#10132=DIRECTION ( 'NONE',  ( -0.000000000000000000, -0.000000000000000000, 1.000000000000000000 ) ) ;
#10134=DIRECTION ( 'NONE',  ( 1.000000000000000000, 0.000000000000000000, 0.000000000000000000 ) ) ;
#10135=DIRECTION ( 'NONE',  ( 0.000000000000000000, 0.000000000000000000, -1.000000000000000000 ) ) ;
#10136=ORIENTED_EDGE ( 'NONE', *, *, #1855, .F. ) ;
#10139=CARTESIAN_POINT ( 'NONE',  ( 2.255998204157473097, -17.85806462366060288, 32.00000000000000000 ) ) ;
#10143=DIRECTION ( 'NONE',  ( 1.000000000000000000, 0.000000000000000000, 0.000000000000000000 ) ) ;
#10145=ADVANCED_FACE ( 'NONE', ( #13057 ), #10644, .F. ) ;
#10150=CARTESIAN_POINT ( 'NONE',  ( 12.86923836996420967, -11.47363181547641453, -32.00000000000000000 ) ) ;
#10154=DIRECTION ( 'NONE',  ( -0.000000000000000000, -0.000000000000000000, 1.000000000000000000 ) ) ;
#10156=CIRCLE ( 'NONE', #15572, 22.00000000000000355 ) ;
#10158=AXIS2_PLACEMENT_3D ( 'NONE', #13436, #16454, #10356 ) ;
#10159=ORIENTED_EDGE ( 'NONE', *, *, #6619, .F. ) ;
#10162=ORIENTED_EDGE ( 'NONE', *, *, #2158, .F. ) ;
#10165=CARTESIAN_POINT ( 'NONE',  ( 13.86923836996420789, -11.47363181547641453, -32.00000000000000000 ) ) ;
#10169=CYLINDRICAL_SURFACE ( 'NONE', #18039, 1.000000000000002665 ) ;
#10177=ORIENTED_EDGE ( 'NONE', *, *, #18687, .T. ) ;
#10179=CARTESIAN_POINT ( 'NONE',  ( -9.671566133830877376, 15.77352024078954429, 32.00000000000000000 ) ) ;
#10189=ADVANCED_FACE ( 'NONE', ( #16550 ), #14849, .F. ) ;
#10194=CARTESIAN_POINT ( 'NONE',  ( -13.86923836996420967, -11.47363181547641275, 35.00000000000000000 ) ) ;
#10199=DIRECTION ( 'NONE',  ( 0.000000000000000000, 0.000000000000000000, -1.000000000000000000 ) ) ;
#10205=CARTESIAN_POINT ( 'NONE',  ( -15.28688694438835505, -7.664027248171298545, -35.00000000000000000 ) ) ;
#10207=EDGE_CURVE ( 'NONE', #226, #257, #17757, .T. ) ;
#10212=LINE ( 'NONE', #3707, #11219 ) ;
#10213=AXIS2_PLACEMENT_3D ( 'NONE', #2244, #11457, #6832 ) ;
#10229=AXIS2_PLACEMENT_3D ( 'NONE', #12116, #4309, #11814 ) ;
#10230=CARTESIAN_POINT ( 'NONE',  ( -18.68117051311639543, -3.372863662543042818, 35.00000000000000000 ) ) ;
#10242=EDGE_CURVE ( 'NONE', #8773, #13907, #9136, .T. ) ;
#10248=ORIENTED_EDGE ( 'NONE', *, *, #15781, .T. ) ;
#10269=CARTESIAN_POINT ( 'NONE',  ( 12.32184790671639618, 13.12143529358541016, 32.00000000000000000 ) ) ;
#10270=AXIS2_PLACEMENT_3D ( 'NONE', #1154, #4349, #5735 ) ;
#10272=DIRECTION ( 'NONE',  ( 0.000000000000000000, 0.000000000000000000, 1.000000000000000000 ) ) ;
#10273=ORIENTED_EDGE ( 'NONE', *, *, #5632, .F. ) ;
#10275=ORIENTED_EDGE ( 'NONE', *, *, #1594, .F. ) ;
#10281=ADVANCED_FACE ( 'NONE', ( #18632 ), #15542, .F. ) ;
#10287=CARTESIAN_POINT ( 'NONE',  ( 2.255998204157473097, -17.85806462366060288, -32.00000000000000000 ) ) ;
#10298=CIRCLE ( 'NONE', #19546, 1.000000000000003553 ) ;
#10306=AXIS2_PLACEMENT_3D ( 'NONE', #1383, #2870, #15184 ) ;
#10308=CARTESIAN_POINT ( 'NONE',  ( 17.11901729331276556, 5.562305898749055011, 32.00000000000000000 ) ) ;
#10322=ORIENTED_EDGE ( 'NONE', *, *, #7570, .T. ) ;
#10323=ADVANCED_FACE ( 'NONE', ( #16465 ), #11852, .F. ) ;
#10326=EDGE_CURVE ( 'NONE', #19705, #1381, #2103, .T. ) ;
#10327=EDGE_CURVE ( 'NONE', #16968, #2987, #16767, .T. ) ;
#10332=DIRECTION ( 'NONE',  ( 0.000000000000000000, 0.000000000000000000, -1.000000000000000000 ) ) ;
#10334=FACE_OUTER_BOUND ( 'NONE', #11084, .T. ) ;
#10335=DIRECTION ( 'NONE',  ( 1.000000000000000000, 0.000000000000000000, 0.000000000000000000 ) ) ;
#10336=ORIENTED_EDGE ( 'NONE', *, *, #8851, .T. ) ;
#10339=DIRECTION ( 'NONE',  ( 0.000000000000000000, 0.000000000000000000, 1.000000000000000000 ) ) ;
#10342=AXIS2_PLACEMENT_3D ( 'NONE', #14763, #12060, #16566 ) ;
#10344=CARTESIAN_POINT ( 'NONE',  ( 0.000000000000000000, 0.000000000000000000, -32.00000000000000000 ) ) ;
#10345=FACE_BOUND ( 'NONE', #14518, .T. ) ;
#10352=AXIS2_PLACEMENT_3D ( 'NONE', #8187, #18790, #18689 ) ;
#10356=DIRECTION ( 'NONE',  ( 1.000000000000000000, 0.000000000000000000, 0.000000000000000000 ) ) ;
#10361=EDGE_LOOP ( 'NONE', ( #1172, #17917 ) ) ;
#10362=VECTOR ( 'NONE', #7614, 1000.000000000000000 ) ;
#10364=LINE ( 'NONE', #7533, #4818 ) ;
#10369=AXIS2_PLACEMENT_3D ( 'NONE', #14066, #473, #12579 ) ;
#10374=ORIENTED_EDGE ( 'NONE', *, *, #12536, .F. ) ;
#10375=EDGE_LOOP ( 'NONE', ( #19132, #16834, #17237, #15660 ) ) ;
#10383=FACE_OUTER_BOUND ( 'NONE', #6268, .T. ) ;
#10392=DIRECTION ( 'NONE',  ( 0.000000000000000000, 0.000000000000000000, 1.000000000000000000 ) ) ;
#10406=CARTESIAN_POINT ( 'NONE',  ( 12.32184790671639618, 13.12143529358541016, -35.00000000000000000 ) ) ;
#10440=ORIENTED_EDGE ( 'NONE', *, *, #11247, .T. ) ;
#10445=CARTESIAN_POINT ( 'NONE',  ( -14.00000000000000178, 0.000000000000000000, -32.00000000000000000 ) ) ;
#10453=CIRCLE ( 'NONE', #12050, 1.000000000000004441 ) ;
#10456=ORIENTED_EDGE ( 'NONE', *, *, #14578, .T. ) ;
#10465=CIRCLE ( 'NONE', #1833, 0.9999999999999974465 ) ;
#10466=ORIENTED_EDGE ( 'NONE', *, *, #2457, .T. ) ;
#10470=VERTEX_POINT ( 'NONE', #1843 ) ;
#10472=DIRECTION ( 'NONE',  ( 1.000000000000000000, 0.000000000000000000, 0.000000000000000000 ) ) ;
#10476=EDGE_CURVE ( 'NONE', #600, #16700, #6885, .T. ) ;
#10477=CARTESIAN_POINT ( 'NONE',  ( -17.28688694438836393, -7.664027248171298545, -35.00000000000000000 ) ) ;
#10480=CARTESIAN_POINT ( 'NONE',  ( 9.671566133830877376, 15.77352024078954784, 35.00000000000000000 ) ) ;
#10483=ADVANCED_FACE ( 'NONE', ( #7014 ), #17452, .F. ) ;
#10490=CARTESIAN_POINT ( 'NONE',  ( -7.626241948324210540, -16.73597674598852336, 32.00000000000000000 ) ) ;
#10493=CARTESIAN_POINT ( 'NONE',  ( 16.28688694438835327, -7.664027248171309203, 32.00000000000000000 ) ) ;
#10496=CARTESIAN_POINT ( 'NONE',  ( -7.626241948324210540, -16.73597674598852336, -32.00000000000000000 ) ) ;
#10499=DIRECTION ( 'NONE',  ( 0.000000000000000000, 0.000000000000000000, 1.000000000000000000 ) ) ;
#10501=LINE ( 'NONE', #7475, #8673 ) ;
#10507=CIRCLE ( 'NONE', #9880, 1.000000000000000888 ) ;
#10508=LINE ( 'NONE', #9002, #6135 ) ;
#10512=FACE_OUTER_BOUND ( 'NONE', #649, .T. ) ;
#10513=CARTESIAN_POINT ( 'NONE',  ( 6.626241948324199882, -16.73597674598852691, 32.00000000000000000 ) ) ;
#10521=AXIS2_PLACEMENT_3D ( 'NONE', #10741, #14306, #17306 ) ;
#10522=CARTESIAN_POINT ( 'NONE',  ( -17.68117051311639898, -3.372863662543042818, -32.00000000000000000 ) ) ;
#10533=LINE ( 'NONE', #18239, #17073 ) ;
#10547=CARTESIAN_POINT ( 'NONE',  ( -22.00000000000000355, 0.000000000000000000, -35.00000000000000000 ) ) ;
#10549=EDGE_CURVE ( 'NONE', #9689, #7585, #4984, .T. ) ;
#10559=FACE_OUTER_BOUND ( 'NONE', #15341, .T. ) ;
#10565=DIRECTION ( 'NONE',  ( 1.000000000000000000, 0.000000000000000000, 0.000000000000000000 ) ) ;
#10567=ORIENTED_EDGE ( 'NONE', *, *, #6736, .F. ) ;
#10569=DIRECTION ( 'NONE',  ( -0.000000000000000000, -0.000000000000000000, 1.000000000000000000 ) ) ;
#10576=ORIENTED_EDGE ( 'NONE', *, *, #1481, .T. ) ;
#10577=DIRECTION ( 'NONE',  ( 0.000000000000000000, 0.000000000000000000, 1.000000000000000000 ) ) ;
#10580=CARTESIAN_POINT ( 'NONE',  ( 3.476417968967386418, 17.43449690031536292, -32.00000000000000000 ) ) ;
#10583=CARTESIAN_POINT ( 'NONE',  ( 14.19790265903627180, 9.644882309621939598, -32.00000000000000000 ) ) ;
#10588=DIRECTION ( 'NONE',  ( 0.000000000000000000, 0.000000000000000000, 1.000000000000000000 ) ) ;
#10593=LINE ( 'NONE', #9194, #1862 ) ;
#10602=DIRECTION ( 'NONE',  ( 1.000000000000000000, 0.000000000000000000, 0.000000000000000000 ) ) ;
#10606=VECTOR ( 'NONE', #2780, 1000.000000000000000 ) ;
#10608=CARTESIAN_POINT ( 'NONE',  ( -17.11901729331276911, 5.562305898749051458, -32.00000000000000000 ) ) ;
#10609=AXIS2_PLACEMENT_3D ( 'NONE', #6810, #5415, #12832 ) ;
#10619=DIRECTION ( 'NONE',  ( 1.000000000000000000, 0.000000000000000000, 0.000000000000000000 ) ) ;
#10623=CIRCLE ( 'NONE', #6437, 0.9999999999999974465 ) ;
#10628=EDGE_CURVE ( 'NONE', #6807, #13831, #12021, .T. ) ;
#10636=VERTEX_POINT ( 'NONE', #1225 ) ;
#10643=CARTESIAN_POINT ( 'NONE',  ( 9.580134541264516912, -14.56230589874905412, 35.00000000000000000 ) ) ;
#10644=CYLINDRICAL_SURFACE ( 'NONE', #18709, 1.000000000000002665 ) ;
#10647=VERTEX_POINT ( 'NONE', #16539 ) ;
#10648=AXIS2_PLACEMENT_3D ( 'NONE', #6170, #19777, #5967 ) ;
#10657=VERTEX_POINT ( 'NONE', #8008 ) ;
#10658=DIRECTION ( 'NONE',  ( 0.000000000000000000, 0.000000000000000000, 1.000000000000000000 ) ) ;
#10661=ORIENTED_EDGE ( 'NONE', *, *, #1956, .F. ) ;
#10662=FACE_OUTER_BOUND ( 'NONE', #19321, .T. ) ;
#10680=DIRECTION ( 'NONE',  ( -0.000000000000000000, -0.000000000000000000, 1.000000000000000000 ) ) ;
#10682=DIRECTION ( 'NONE',  ( 0.000000000000000000, 0.000000000000000000, 1.000000000000000000 ) ) ;
#10691=DIRECTION ( 'NONE',  ( -0.000000000000000000, -0.000000000000000000, 1.000000000000000000 ) ) ;
#10693=CIRCLE ( 'NONE', #10066, 1.000000000000004441 ) ;
#10705=ORIENTED_EDGE ( 'NONE', *, *, #9812, .T. ) ;
#10706=AXIS2_PLACEMENT_3D ( 'NONE', #5639, #8747, #16353 ) ;
#10715=CYLINDRICAL_SURFACE ( 'NONE', #1192, 1.000000000000004441 ) ;
#10716=ORIENTED_EDGE ( 'NONE', *, *, #6565, .F. ) ;
#10718=CARTESIAN_POINT ( 'NONE',  ( -12.86923836996420611, -11.47363181547641275, -35.00000000000000000 ) ) ;
#10720=ADVANCED_FACE ( 'NONE', ( #3215 ), #13829, .F. ) ;
#10737=ADVANCED_FACE ( 'NONE', ( #6498 ), #6596, .F. ) ;
#10738=DIRECTION ( 'NONE',  ( 1.000000000000000000, 0.000000000000000000, 0.000000000000000000 ) ) ;
#10741=CARTESIAN_POINT ( 'NONE',  ( -2.255998204157477538, -17.85806462366060288, -32.00000000000000000 ) ) ;
#10747=AXIS2_PLACEMENT_3D ( 'NONE', #8608, #10029, #912 ) ;
#10764=CARTESIAN_POINT ( 'NONE',  ( 4.476417968967386862, 17.43449690031536292, -35.00000000000000000 ) ) ;
#10766=ORIENTED_EDGE ( 'NONE', *, *, #14108, .F. ) ;
#10768=ADVANCED_FACE ( 'NONE', ( #9231 ), #12333, .F. ) ;
#10773=AXIS2_PLACEMENT_3D ( 'NONE', #1116, #7189, #6904 ) ;
#10785=FACE_BOUND ( 'NONE', #5261, .T. ) ;
#10789=VECTOR ( 'NONE', #14159, 1000.000000000000000 ) ;
#10790=VERTEX_POINT ( 'NONE', #12528 ) ;
#10792=CARTESIAN_POINT ( 'NONE',  ( 16.19790265903627358, 9.644882309621939598, -32.00000000000000000 ) ) ;
#10793=ORIENTED_EDGE ( 'NONE', *, *, #5543, .F. ) ;
#10800=ORIENTED_EDGE ( 'NONE', *, *, #2231, .T. ) ;
#10804=FACE_OUTER_BOUND ( 'NONE', #7040, .T. ) ;
#10805=VECTOR ( 'NONE', #11920, 1000.000000000000000 ) ;
#10820=AXIS2_PLACEMENT_3D ( 'NONE', #3969, #13074, #6653 ) ;
#10826=DIRECTION ( 'NONE',  ( 0.000000000000000000, 0.000000000000000000, 1.000000000000000000 ) ) ;
#10827=DIRECTION ( 'NONE',  ( -0.000000000000000000, -0.000000000000000000, -1.000000000000000000 ) ) ;
#10828=EDGE_CURVE ( 'NONE', #11862, #13666, #17322, .T. ) ;
#10844=CYLINDRICAL_SURFACE ( 'NONE', #3672, 1.000000000000000888 ) ;
#10850=ORIENTED_EDGE ( 'NONE', *, *, #12607, .T. ) ;
#10852=FACE_OUTER_BOUND ( 'NONE', #10375, .T. ) ;
#10856=VERTEX_POINT ( 'NONE', #14716 ) ;
#10861=ORIENTED_EDGE ( 'NONE', *, *, #3515, .F. ) ;
#10864=EDGE_CURVE ( 'NONE', #19421, #9729, #12350, .T. ) ;
#10867=CARTESIAN_POINT ( 'NONE',  ( 17.68117051311639898, -3.372863662543048591, -32.00000000000000000 ) ) ;
#10872=EDGE_CURVE ( 'NONE', #18625, #5897, #14424, .T. ) ;
#10876=ORIENTED_EDGE ( 'NONE', *, *, #8826, .F. ) ;
#10879=AXIS2_PLACEMENT_3D ( 'NONE', #13220, #15113, #8708 ) ;
#10885=DIRECTION ( 'NONE',  ( 1.000000000000000000, 0.000000000000000000, 0.000000000000000000 ) ) ;
#10886=EDGE_CURVE ( 'NONE', #1540, #17520, #5211, .T. ) ;
#10890=CARTESIAN_POINT ( 'NONE',  ( 7.626241948324204323, -16.73597674598852691, 35.00000000000000000 ) ) ;
#10891=CARTESIAN_POINT ( 'NONE',  ( 15.19790265903627358, 9.644882309621939598, -32.00000000000000000 ) ) ;
#10895=CIRCLE ( 'NONE', #5759, 1.000000000000002442 ) ;
#10897=DIRECTION ( 'NONE',  ( -0.000000000000000000, -0.000000000000000000, 1.000000000000000000 ) ) ;
#10900=VERTEX_POINT ( 'NONE', #16220 ) ;
#10911=EDGE_LOOP ( 'NONE', ( #11243, #5255 ) ) ;
#10913=DIRECTION ( 'NONE',  ( -0.000000000000000000, -0.000000000000000000, -1.000000000000000000 ) ) ;
#10915=ORIENTED_EDGE ( 'NONE', *, *, #13709, .T. ) ;
#10919=EDGE_CURVE ( 'NONE', #7633, #15498, #17772, .T. ) ;
#10921=CIRCLE ( 'NONE', #7727, 1.000000000000003109 ) ;
#10928=CYLINDRICAL_SURFACE ( 'NONE', #9422, 14.00000000000000178 ) ;
#10935=DIRECTION ( 'NONE',  ( 1.000000000000000000, 0.000000000000000000, 0.000000000000000000 ) ) ;
#10954=ORIENTED_EDGE ( 'NONE', *, *, #9669, .F. ) ;
#10957=VECTOR ( 'NONE', #11145, 1000.000000000000000 ) ;
#10968=DIRECTION ( 'NONE',  ( 1.000000000000000000, 0.000000000000000000, 0.000000000000000000 ) ) ;
#10975=FACE_BOUND ( 'NONE', #14238, .T. ) ;
#10978=CARTESIAN_POINT ( 'NONE',  ( -16.28688694438836038, -7.664027248171298545, 32.00000000000000000 ) ) ;
#10979=VERTEX_POINT ( 'NONE', #7486 ) ;
#10980=EDGE_LOOP ( 'NONE', ( #12713, #8937, #3951, #13344 ) ) ;
#10984=CARTESIAN_POINT ( 'NONE',  ( -18.96448111170889206, 1.130229351527647808, 32.00000000000000000 ) ) ;
#10995=CYLINDRICAL_SURFACE ( 'NONE', #388, 0.9999999999999974465 ) ;
#11000=DIRECTION ( 'NONE',  ( -0.000000000000000000, -0.000000000000000000, 1.000000000000000000 ) ) ;
#11002=ORIENTED_EDGE ( 'NONE', *, *, #4599, .T. ) ;
#11003=CARTESIAN_POINT ( 'NONE',  ( -15.28688694438835505, -7.664027248171298545, -32.00000000000000000 ) ) ;
#11006=DIRECTION ( 'NONE',  ( 1.000000000000000000, 0.000000000000000000, 0.000000000000000000 ) ) ;
#11015=EDGE_CURVE ( 'NONE', #271, #10979, #219, .T. ) ;
#11028=CARTESIAN_POINT ( 'NONE',  ( 5.476417968967387750, 17.43449690031536292, 32.00000000000000000 ) ) ;
#11031=ORIENTED_EDGE ( 'NONE', *, *, #9558, .T. ) ;
#11032=CARTESIAN_POINT ( 'NONE',  ( -4.476417968967385974, 17.43449690031536292, -32.00000000000000000 ) ) ;
#11033=DIRECTION ( 'NONE',  ( 0.000000000000000000, 0.000000000000000000, -1.000000000000000000 ) ) ;
#11041=ORIENTED_EDGE ( 'NONE', *, *, #13948, .T. ) ;
#11046=ORIENTED_EDGE ( 'NONE', *, *, #2897, .F. ) ;
#11058=ORIENTED_EDGE ( 'NONE', *, *, #14767, .F. ) ;
#11070=DIRECTION ( 'NONE',  ( -0.000000000000000000, -0.000000000000000000, 1.000000000000000000 ) ) ;
#11081=CARTESIAN_POINT ( 'NONE',  ( 9.580134541264516912, -14.56230589874905412, -35.00000000000000000 ) ) ;
#11083=ADVANCED_FACE ( 'NONE', ( #15697 ), #15603, .F. ) ;
#11084=EDGE_LOOP ( 'NONE', ( #10456, #11169, #11377, #19330 ) ) ;
#11086=CARTESIAN_POINT ( 'NONE',  ( -17.11901729331276911, 5.562305898749051458, -35.00000000000000000 ) ) ;
#11088=ORIENTED_EDGE ( 'NONE', *, *, #6861, .T. ) ;
#11091=FACE_OUTER_BOUND ( 'NONE', #342, .T. ) ;
#11093=DIRECTION ( 'NONE',  ( 1.000000000000000000, 0.000000000000000000, 0.000000000000000000 ) ) ;
#11099=CYLINDRICAL_SURFACE ( 'NONE', #9756, 0.9999999999999974465 ) ;
#11109=DIRECTION ( 'NONE',  ( 1.000000000000000000, 0.000000000000000000, 0.000000000000000000 ) ) ;
#11111=DIRECTION ( 'NONE',  ( 0.000000000000000000, 0.000000000000000000, -1.000000000000000000 ) ) ;
#11112=EDGE_CURVE ( 'NONE', #6062, #16380, #12309, .T. ) ;
#11115=CARTESIAN_POINT ( 'NONE',  ( 10.58013454126452046, -14.56230589874905412, -32.00000000000000000 ) ) ;
#11117=CIRCLE ( 'NONE', #5043, 1.000000000000002665 ) ;
#11118=CIRCLE ( 'NONE', #15920, 0.9999999999999974465 ) ;
#11121=ORIENTED_EDGE ( 'NONE', *, *, #2266, .T. ) ;
#11126=EDGE_LOOP ( 'NONE', ( #711, #9780, #16025, #19435 ) ) ;
#11136=AXIS2_PLACEMENT_3D ( 'NONE', #4363, #4066, #8768 ) ;
#11138=EDGE_CURVE ( 'NONE', #13907, #8773, #16519, .T. ) ;
#11139=ADVANCED_FACE ( 'NONE', ( #3396 ), #15994, .F. ) ;
#11145=DIRECTION ( 'NONE',  ( 0.000000000000000000, 0.000000000000000000, 1.000000000000000000 ) ) ;
#11146=DIRECTION ( 'NONE',  ( 1.000000000000000000, 0.000000000000000000, 0.000000000000000000 ) ) ;
#11149=EDGE_LOOP ( 'NONE', ( #8973, #11977, #1643, #13622 ) ) ;
#11152=ORIENTED_EDGE ( 'NONE', *, *, #16598, .T. ) ;
#11155=ORIENTED_EDGE ( 'NONE', *, *, #12322, .T. ) ;
#11164=ORIENTED_EDGE ( 'NONE', *, *, #9015, .F. ) ;
#11166=EDGE_CURVE ( 'NONE', #9602, #7536, #18994, .T. ) ;
#11169=ORIENTED_EDGE ( 'NONE', *, *, #4174, .T. ) ;
#11173=DIRECTION ( 'NONE',  ( 1.000000000000000000, 0.000000000000000000, 0.000000000000000000 ) ) ;
#11174=ORIENTED_EDGE ( 'NONE', *, *, #6619, .T. ) ;
#11179=ORIENTED_EDGE ( 'NONE', *, *, #13484, .F. ) ;
#11187=VERTEX_POINT ( 'NONE', #888 ) ;
#11193=DIRECTION ( 'NONE',  ( -1.000000000000000000, 0.000000000000000000, 0.000000000000000000 ) ) ;
#11196=DIRECTION ( 'NONE',  ( 0.000000000000000000, 0.000000000000000000, -1.000000000000000000 ) ) ;
#11199=ORIENTED_EDGE ( 'NONE', *, *, #15781, .F. ) ;
#11219=VECTOR ( 'NONE', #11702, 1000.000000000000000 ) ;
#11224=ORIENTED_EDGE ( 'NONE', *, *, #15296, .F. ) ;
#11236=AXIS2_PLACEMENT_3D ( 'NONE', #14142, #9857, #18841 ) ;
#11240=CYLINDRICAL_SURFACE ( 'NONE', #19254, 1.000000000000000000 ) ;
#11243=ORIENTED_EDGE ( 'NONE', *, *, #11379, .T. ) ;
#11247=EDGE_CURVE ( 'NONE', #12336, #6290, #1805, .T. ) ;
#11248=EDGE_LOOP ( 'NONE', ( #1024, #11088, #17982, #15008 ) ) ;
#11258=DIRECTION ( 'NONE',  ( 0.000000000000000000, 0.000000000000000000, -1.000000000000000000 ) ) ;
#11259=CYLINDRICAL_SURFACE ( 'NONE', #8554, 0.9999999999999974465 ) ;
#11272=CARTESIAN_POINT ( 'NONE',  ( 4.476417968967386862, 17.43449690031536292, -32.00000000000000000 ) ) ;
#11273=EDGE_CURVE ( 'NONE', #8799, #676, #19087, .T. ) ;
#11282=EDGE_CURVE ( 'NONE', #4912, #6438, #17784, .T. ) ;
#11286=ORIENTED_EDGE ( 'NONE', *, *, #16462, .F. ) ;
#11287=DIRECTION ( 'NONE',  ( 0.000000000000000000, 0.000000000000000000, 1.000000000000000000 ) ) ;
#11290=ORIENTED_EDGE ( 'NONE', *, *, #13059, .F. ) ;
#11292=ADVANCED_FACE ( 'NONE', ( #3785 ), #597, .F. ) ;
#11302=CIRCLE ( 'NONE', #13536, 0.9999999999999974465 ) ;
#11304=VERTEX_POINT ( 'NONE', #5962 ) ;
#11308=EDGE_CURVE ( 'NONE', #3152, #13990, #8981, .T. ) ;
#11311=VERTEX_POINT ( 'NONE', #11881 ) ;
#11319=EDGE_LOOP ( 'NONE', ( #5196, #19458, #14967, #16942 ) ) ;
#11326=ORIENTED_EDGE ( 'NONE', *, *, #2785, .T. ) ;
#11336=VERTEX_POINT ( 'NONE', #8680 ) ;
#11339=DIRECTION ( 'NONE',  ( 0.000000000000000000, 0.000000000000000000, 1.000000000000000000 ) ) ;
#11348=AXIS2_PLACEMENT_3D ( 'NONE', #12408, #3296, #2087 ) ;
#11351=EDGE_LOOP ( 'NONE', ( #18212, #13072, #7543, #18216 ) ) ;
#11370=ORIENTED_EDGE ( 'NONE', *, *, #17394, .T. ) ;
#11371=CIRCLE ( 'NONE', #19033, 1.000000000000003109 ) ;
#11377=ORIENTED_EDGE ( 'NONE', *, *, #16487, .F. ) ;
#11379=EDGE_CURVE ( 'NONE', #1540, #7513, #10465, .T. ) ;
#11380=ORIENTED_EDGE ( 'NONE', *, *, #1920, .F. ) ;
#11381=CARTESIAN_POINT ( 'NONE',  ( -8.671566133830875600, 15.77352024078954429, 32.00000000000000000 ) ) ;
#11391=AXIS2_PLACEMENT_3D ( 'NONE', #620, #6696, #18917 ) ;
#11393=DIRECTION ( 'NONE',  ( 1.000000000000000000, 0.000000000000000000, -0.000000000000000000 ) ) ;
#11396=DIRECTION ( 'NONE',  ( 0.000000000000000000, 0.000000000000000000, 1.000000000000000000 ) ) ;
#11400=DIRECTION ( 'NONE',  ( 1.000000000000000000, 0.000000000000000000, 0.000000000000000000 ) ) ;
#11404=CARTESIAN_POINT ( 'NONE',  ( 11.32184790671639263, 13.12143529358541016, 35.00000000000000000 ) ) ;
#11407=VECTOR ( 'NONE', #12831, 1000.000000000000000 ) ;
#11409=EDGE_CURVE ( 'NONE', #15039, #15498, #16491, .T. ) ;
#11415=DIRECTION ( 'NONE',  ( 0.000000000000000000, 0.000000000000000000, -1.000000000000000000 ) ) ;
#11420=EDGE_LOOP ( 'NONE', ( #17469, #6686, #6613, #13042 ) ) ;
#11429=DIRECTION ( 'NONE',  ( 0.000000000000000000, 0.000000000000000000, 1.000000000000000000 ) ) ;
#11435=DIRECTION ( 'NONE',  ( 0.000000000000000000, 0.000000000000000000, 1.000000000000000000 ) ) ;
#11440=CIRCLE ( 'NONE', #11747, 1.000000000000002665 ) ;
#11441=ORIENTED_EDGE ( 'NONE', *, *, #286, .T. ) ;
#11447=DIRECTION ( 'NONE',  ( 0.000000000000000000, 0.000000000000000000, -1.000000000000000000 ) ) ;
#11457=DIRECTION ( 'NONE',  ( 0.000000000000000000, 0.000000000000000000, 1.000000000000000000 ) ) ;
#11462=DIRECTION ( 'NONE',  ( 0.000000000000000000, 0.000000000000000000, 1.000000000000000000 ) ) ;
#11463=DIRECTION ( 'NONE',  ( 1.000000000000000000, 0.000000000000000000, 0.000000000000000000 ) ) ;
#11475=ORIENTED_EDGE ( 'NONE', *, *, #11653, .T. ) ;
#11476=VERTEX_POINT ( 'NONE', #7861 ) ;
#11479=DIRECTION ( 'NONE',  ( 0.000000000000000000, 0.000000000000000000, 1.000000000000000000 ) ) ;
#11481=DIRECTION ( 'NONE',  ( 1.000000000000000000, 0.000000000000000000, 0.000000000000000000 ) ) ;
#11492=DIRECTION ( 'NONE',  ( 0.000000000000000000, 0.000000000000000000, 1.000000000000000000 ) ) ;
#11493=CARTESIAN_POINT ( 'NONE',  ( 18.96448111170889206, 1.130229351527639148, 32.00000000000000000 ) ) ;
#11494=EDGE_CURVE ( 'NONE', #19430, #4232, #6446, .T. ) ;
#11495=CARTESIAN_POINT ( 'NONE',  ( -5.476417968967388639, 17.43449690031536292, 32.00000000000000000 ) ) ;
#11501=CYLINDRICAL_SURFACE ( 'NONE', #17985, 1.000000000000004441 ) ;
#11514=ORIENTED_EDGE ( 'NONE', *, *, #9981, .T. ) ;
#11520=CARTESIAN_POINT ( 'NONE',  ( 4.476417968967386862, 17.43449690031536292, 32.00000000000000000 ) ) ;
#11521=EDGE_LOOP ( 'NONE', ( #19231, #18180, #474, #3704 ) ) ;
#11522=CIRCLE ( 'NONE', #5112, 1.000000000000000888 ) ;
#11525=DIRECTION ( 'NONE',  ( 1.000000000000000000, 0.000000000000000000, 0.000000000000000000 ) ) ;
#11527=VERTEX_POINT ( 'NONE', #362 ) ;
#11528=FACE_BOUND ( 'NONE', #6211, .T. ) ;
#11529=EDGE_CURVE ( 'NONE', #6632, #3405, #3370, .T. ) ;
#11531=DIRECTION ( 'NONE',  ( 1.000000000000000000, 0.000000000000000000, 0.000000000000000000 ) ) ;
#11540=CARTESIAN_POINT ( 'NONE',  ( 14.86923836996420434, -11.47363181547641453, 32.00000000000000000 ) ) ;
#11547=LINE ( 'NONE', #17653, #11556 ) ;
#11550=DIRECTION ( 'NONE',  ( 0.000000000000000000, 0.000000000000000000, -1.000000000000000000 ) ) ;
#11551=CARTESIAN_POINT ( 'NONE',  ( -3.255998204157480203, -17.85806462366060288, 35.00000000000000000 ) ) ;
#11553=AXIS2_PLACEMENT_3D ( 'NONE', #14337, #5120, #8439 ) ;
#11556=VECTOR ( 'NONE', #14657, 1000.000000000000000 ) ;
#11559=CIRCLE ( 'NONE', #15077, 0.9999999999999974465 ) ;
#11567=AXIS2_PLACEMENT_3D ( 'NONE', #10194, #18996, #15995 ) ;
#11568=EDGE_LOOP ( 'NONE', ( #556, #12676 ) ) ;
#11571=DIRECTION ( 'NONE',  ( 0.000000000000000000, 0.000000000000000000, -1.000000000000000000 ) ) ;
#11572=AXIS2_PLACEMENT_3D ( 'NONE', #9706, #4986, #13999 ) ;
#11575=ORIENTED_EDGE ( 'NONE', *, *, #18526, .F. ) ;
#11579=ORIENTED_EDGE ( 'NONE', *, *, #14767, .T. ) ;
#11586=CIRCLE ( 'NONE', #19251, 1.000000000000000888 ) ;
#11590=CIRCLE ( 'NONE', #5514, 1.000000000000004441 ) ;
#11591=ORIENTED_EDGE ( 'NONE', *, *, #4757, .F. ) ;
#11595=UNCERTAINTY_MEASURE_WITH_UNIT (LENGTH_MEASURE( 1.000000000000000082E-05 ), #4650, 'distance_accuracy_value', 'NONE');
#11600=DIRECTION ( 'NONE',  ( 0.000000000000000000, 0.000000000000000000, -1.000000000000000000 ) ) ;
#11604=EDGE_CURVE ( 'NONE', #6062, #11862, #10453, .T. ) ;
#11610=ORIENTED_EDGE ( 'NONE', *, *, #11657, .T. ) ;
#11612=CARTESIAN_POINT ( 'NONE',  ( 17.96448111170888851, 1.130229351527639148, 32.00000000000000000 ) ) ;
#11616=ORIENTED_EDGE ( 'NONE', *, *, #4757, .T. ) ;
#11618=DIRECTION ( 'NONE',  ( 0.000000000000000000, 0.000000000000000000, -1.000000000000000000 ) ) ;
#11627=ORIENTED_EDGE ( 'NONE', *, *, #10919, .F. ) ;
#11628=EDGE_CURVE ( 'NONE', #8576, #11336, #19707, .T. ) ;
#11636=FACE_BOUND ( 'NONE', #19142, .T. ) ;
#11653=EDGE_CURVE ( 'NONE', #10856, #7344, #18872, .T. ) ;
#11655=VERTEX_POINT ( 'NONE', #3468 ) ;
#11656=DIRECTION ( 'NONE',  ( 1.000000000000000000, 0.000000000000000000, 0.000000000000000000 ) ) ;
#11657=EDGE_CURVE ( 'NONE', #3117, #8877, #13645, .T. ) ;
#11665=CARTESIAN_POINT ( 'NONE',  ( 8.671566133830875600, 15.77352024078954784, -32.00000000000000000 ) ) ;
#11666=EDGE_CURVE ( 'NONE', #3037, #9666, #674, .T. ) ;
#11670=AXIS2_PLACEMENT_3D ( 'NONE', #12963, #15963, #855 ) ;
#11671=CARTESIAN_POINT ( 'NONE',  ( 14.19790265903627180, 9.644882309621939598, -32.00000000000000000 ) ) ;
#11672=AXIS2_PLACEMENT_3D ( 'NONE', #8083, #18891, #18593 ) ;
#11682=AXIS2_PLACEMENT_3D ( 'NONE', #28, #14131, #4829 ) ;
#11683=DIRECTION ( 'NONE',  ( 0.000000000000000000, 0.000000000000000000, -1.000000000000000000 ) ) ;
#11685=VECTOR ( 'NONE', #11479, 1000.000000000000000 ) ;
#11688=DIRECTION ( 'NONE',  ( -1.000000000000000000, 0.000000000000000000, 0.000000000000000000 ) ) ;
#11690=CARTESIAN_POINT ( 'NONE',  ( 1.000000000000003331, 18.00000000000000355, 32.00000000000000000 ) ) ;
#11695=VERTEX_POINT ( 'NONE', #17743 ) ;
#11697=AXIS2_PLACEMENT_3D ( 'NONE', #18426, #1724, #7814 ) ;
#11699=DIRECTION ( 'NONE',  ( 0.000000000000000000, 0.000000000000000000, -1.000000000000000000 ) ) ;
#11702=DIRECTION ( 'NONE',  ( 0.000000000000000000, 0.000000000000000000, 1.000000000000000000 ) ) ;
#11708=DIRECTION ( 'NONE',  ( 1.000000000000000000, 0.000000000000000000, 0.000000000000000000 ) ) ;
#11725=AXIS2_PLACEMENT_3D ( 'NONE', #13334, #14374, #2163 ) ;
#11727=AXIS2_PLACEMENT_3D ( 'NONE', #2411, #11618, #13124 ) ;
#11731=EDGE_LOOP ( 'NONE', ( #9577, #11475, #17214, #14315 ) ) ;
#11736=CARTESIAN_POINT ( 'NONE',  ( 1.000000000000003331, 18.00000000000000355, -35.00000000000000000 ) ) ;
#11737=ORIENTED_EDGE ( 'NONE', *, *, #3560, .T. ) ;
#11747=AXIS2_PLACEMENT_3D ( 'NONE', #4209, #6090, #2796 ) ;
#11750=EDGE_LOOP ( 'NONE', ( #1095, #5728 ) ) ;
#11751=CARTESIAN_POINT ( 'NONE',  ( 11.32184790671639263, 13.12143529358541016, -32.00000000000000000 ) ) ;
#11754=CYLINDRICAL_SURFACE ( 'NONE', #9646, 1.000000000000004441 ) ;
#11765=VERTEX_POINT ( 'NONE', #16845 ) ;
#11767=DIRECTION ( 'NONE',  ( 0.000000000000000000, 0.000000000000000000, -1.000000000000000000 ) ) ;
#11769=ORIENTED_EDGE ( 'NONE', *, *, #18131, .T. ) ;
#11772=ORIENTED_EDGE ( 'NONE', *, *, #18962, .T. ) ;
#11773=DIRECTION ( 'NONE',  ( 1.000000000000000000, 0.000000000000000000, 0.000000000000000000 ) ) ;
#11774=EDGE_CURVE ( 'NONE', #16239, #18193, #3124, .T. ) ;
#11779=EDGE_CURVE ( 'NONE', #2901, #2678, #8214, .T. ) ;
#11804=DIRECTION ( 'NONE',  ( -0.000000000000000000, -0.000000000000000000, 1.000000000000000000 ) ) ;
#11806=ORIENTED_EDGE ( 'NONE', *, *, #5175, .T. ) ;
#11810=CARTESIAN_POINT ( 'NONE',  ( -22.00000000000000355, 2.694222958124177204E-15, 32.00000000000000000 ) ) ;
#11811=VERTEX_POINT ( 'NONE', #12041 ) ;
#11812=CARTESIAN_POINT ( 'NONE',  ( 0.000000000000000000, 0.000000000000000000, -32.00000000000000000 ) ) ;
#11814=DIRECTION ( 'NONE',  ( 1.000000000000000000, 0.000000000000000000, 0.000000000000000000 ) ) ;
#11822=ORIENTED_EDGE ( 'NONE', *, *, #12286, .F. ) ;
#11825=CARTESIAN_POINT ( 'NONE',  ( 12.32184790671639618, 13.12143529358541016, -32.00000000000000000 ) ) ;
#11827=VERTEX_POINT ( 'NONE', #18336 ) ;
#11828=VECTOR ( 'NONE', #10199, 1000.000000000000000 ) ;
#11832=FACE_BOUND ( 'NONE', #3564, .T. ) ;
#11841=DIRECTION ( 'NONE',  ( -1.000000000000000000, 0.000000000000000000, 0.000000000000000000 ) ) ;
#11843=ORIENTED_EDGE ( 'NONE', *, *, #14921, .T. ) ;
#11852=CYLINDRICAL_SURFACE ( 'NONE', #13933, 1.000000000000002665 ) ;
#11856=VECTOR ( 'NONE', #13549, 1000.000000000000000 ) ;
#11857=EDGE_LOOP ( 'NONE', ( #8372, #15640, #8464, #14816 ) ) ;
#11862=VERTEX_POINT ( 'NONE', #1329 ) ;
#11869=EDGE_LOOP ( 'NONE', ( #10716, #3323 ) ) ;
#11872=ADVANCED_FACE ( 'NONE', ( #7718 ), #5720, .F. ) ;
#11874=ORIENTED_EDGE ( 'NONE', *, *, #8779, .F. ) ;
#11881=CARTESIAN_POINT ( 'NONE',  ( 3.476417968967386418, 17.43449690031536292, 35.00000000000000000 ) ) ;
#11887=FACE_BOUND ( 'NONE', #9004, .T. ) ;
#11889=CARTESIAN_POINT ( 'NONE',  ( -12.32184790671639085, 13.12143529358541549, -35.00000000000000000 ) ) ;
#11904=CARTESIAN_POINT ( 'NONE',  ( 13.86923836996420789, -11.47363181547641453, 35.00000000000000000 ) ) ;
#11905=ORIENTED_EDGE ( 'NONE', *, *, #9558, .F. ) ;
#11907=CARTESIAN_POINT ( 'NONE',  ( 15.19790265903627358, 9.644882309621939598, 32.00000000000000000 ) ) ;
#11911=CIRCLE ( 'NONE', #13185, 1.000000000000000888 ) ;
#11920=DIRECTION ( 'NONE',  ( 0.000000000000000000, 0.000000000000000000, -1.000000000000000000 ) ) ;
#11928=EDGE_LOOP ( 'NONE', ( #8424, #15177 ) ) ;
#11937=ORIENTED_EDGE ( 'NONE', *, *, #13174, .T. ) ;
#11940=CARTESIAN_POINT ( 'NONE',  ( -8.671566133830875600, 15.77352024078954429, 32.00000000000000000 ) ) ;
#11949=PRODUCT_DEFINITION_SHAPE ( 'NONE', 'NONE',  #8823 ) ;
#11951=EDGE_CURVE ( 'NONE', #2783, #17931, #9852, .T. ) ;
#11955=DIRECTION ( 'NONE',  ( 0.000000000000000000, 0.000000000000000000, -1.000000000000000000 ) ) ;
#11958=ORIENTED_EDGE ( 'NONE', *, *, #19165, .F. ) ;
#11959=LINE ( 'NONE', #2743, #19625 ) ;
#11960=CIRCLE ( 'NONE', #3336, 1.000000000000004441 ) ;
#11973=ORIENTED_EDGE ( 'NONE', *, *, #19384, .F. ) ;
#11977=ORIENTED_EDGE ( 'NONE', *, *, #1500, .T. ) ;
#11985=CYLINDRICAL_SURFACE ( 'NONE', #3262, 1.000000000000004441 ) ;
#11986=ORIENTED_EDGE ( 'NONE', *, *, #7969, .T. ) ;
#11987=DIRECTION ( 'NONE',  ( 1.000000000000000000, 0.000000000000000000, 0.000000000000000000 ) ) ;
#11991=VECTOR ( 'NONE', #14647, 1000.000000000000000 ) ;
#11993=EDGE_CURVE ( 'NONE', #17321, #14722, #2790, .T. ) ;
#12007=ORIENTED_EDGE ( 'NONE', *, *, #14616, .T. ) ;
#12010=DIRECTION ( 'NONE',  ( 1.000000000000000000, 0.000000000000000000, 0.000000000000000000 ) ) ;
#12017=CARTESIAN_POINT ( 'NONE',  ( 6.626241948324199882, -16.73597674598852691, 32.00000000000000000 ) ) ;
#12021=CIRCLE ( 'NONE', #4672, 14.00000000000000178 ) ;
#12024=ORIENTED_EDGE ( 'NONE', *, *, #7953, .F. ) ;
#12040=ORIENTED_EDGE ( 'NONE', *, *, #15945, .F. ) ;
#12041=CARTESIAN_POINT ( 'NONE',  ( -18.11901729331277267, 5.562305898749051458, -32.00000000000000000 ) ) ;
#12044=LINE ( 'NONE', #1436, #15708 ) ;
#12048=VERTEX_POINT ( 'NONE', #424 ) ;
#12049=CARTESIAN_POINT ( 'NONE',  ( 2.255998204157473097, -17.85806462366060288, -32.00000000000000000 ) ) ;
#12050=AXIS2_PLACEMENT_3D ( 'NONE', #17080, #12284, #1868 ) ;
#12060=DIRECTION ( 'NONE',  ( 0.000000000000000000, 0.000000000000000000, 1.000000000000000000 ) ) ;
#12064=ORIENTED_EDGE ( 'NONE', *, *, #17036, .T. ) ;
#12071=DIRECTION ( 'NONE',  ( 1.000000000000000000, 0.000000000000000000, 0.000000000000000000 ) ) ;
#12076=LINE ( 'NONE', #7653, #1036 ) ;
#12086=ORIENTED_EDGE ( 'NONE', *, *, #14578, .F. ) ;
#12090=DIRECTION ( 'NONE',  ( 1.000000000000000000, 0.000000000000000000, 0.000000000000000000 ) ) ;
#12092=PLANE ( 'NONE',  #6599 ) ;
#12096=FACE_OUTER_BOUND ( 'NONE', #8886, .T. ) ;
#12099=EDGE_CURVE ( 'NONE', #9666, #1561, #18130, .T. ) ;
#12104=CIRCLE ( 'NONE', #4116, 1.000000000000002665 ) ;
#12105=ADVANCED_FACE ( 'NONE', ( #6703 ), #12827, .F. ) ;
#12106=DIRECTION ( 'NONE',  ( -0.000000000000000000, -0.000000000000000000, 1.000000000000000000 ) ) ;
#12110=DIRECTION ( 'NONE',  ( -0.000000000000000000, -0.000000000000000000, 1.000000000000000000 ) ) ;
#12114=FACE_OUTER_BOUND ( 'NONE', #19417, .T. ) ;
#12116=CARTESIAN_POINT ( 'NONE',  ( 17.96448111170888851, 1.130229351527639148, -35.00000000000000000 ) ) ;
#12117=DIRECTION ( 'NONE',  ( 1.000000000000000000, 0.000000000000000000, 0.000000000000000000 ) ) ;
#12118=DIRECTION ( 'NONE',  ( -1.000000000000000000, 0.000000000000000000, 0.000000000000000000 ) ) ;
#12121=CARTESIAN_POINT ( 'NONE',  ( 4.476417968967386862, 17.43449690031536292, -32.00000000000000000 ) ) ;
#12122=ORIENTED_EDGE ( 'NONE', *, *, #2356, .F. ) ;
#12131=VERTEX_POINT ( 'NONE', #16026 ) ;
#12135=CARTESIAN_POINT ( 'NONE',  ( 5.476417968967387750, 17.43449690031536292, 32.00000000000000000 ) ) ;
#12149=CARTESIAN_POINT ( 'NONE',  ( 18.68117051311639543, -3.372863662543048591, -32.00000000000000000 ) ) ;
#12151=CIRCLE ( 'NONE', #16617, 0.9999999999999974465 ) ;
#12152=ORIENTED_EDGE ( 'NONE', *, *, #2731, .T. ) ;
#12163=CARTESIAN_POINT ( 'NONE',  ( -15.19790265903627180, 9.644882309621941374, 32.00000000000000000 ) ) ;
#12165=EDGE_CURVE ( 'NONE', #11862, #6062, #15266, .T. ) ;
#12167=EDGE_LOOP ( 'NONE', ( #13596, #15165 ) ) ;
#12178=CARTESIAN_POINT ( 'NONE',  ( 10.58013454126452046, -14.56230589874905412, -35.00000000000000000 ) ) ;
#12182=EDGE_CURVE ( 'NONE', #16673, #11527, #1847, .T. ) ;
#12188=AXIS2_PLACEMENT_3D ( 'NONE', #6416, #5036, #9652 ) ;
#12196=EDGE_LOOP ( 'NONE', ( #11627, #13437 ) ) ;
#12216=ORIENTED_EDGE ( 'NONE', *, *, #15945, .T. ) ;
#12217=DIRECTION ( 'NONE',  ( 1.000000000000000000, 0.000000000000000000, 0.000000000000000000 ) ) ;
#12224=AXIS2_PLACEMENT_3D ( 'NONE', #17004, #792, #6864 ) ;
#12225=VERTEX_POINT ( 'NONE', #9011 ) ;
#12226=AXIS2_PLACEMENT_3D ( 'NONE', #13768, #10577, #6246 ) ;
#12229=CARTESIAN_POINT ( 'NONE',  ( -16.96448111170888851, 1.130229351527647808, -35.00000000000000000 ) ) ;
#12235=ORIENTED_EDGE ( 'NONE', *, *, #1125, .T. ) ;
#12262=DIRECTION ( 'NONE',  ( 1.000000000000000000, 0.000000000000000000, 0.000000000000000000 ) ) ;
#12263=DIRECTION ( 'NONE',  ( 1.000000000000000000, 0.000000000000000000, 0.000000000000000000 ) ) ;
#12264=ORIENTED_EDGE ( 'NONE', *, *, #15178, .T. ) ;
#12276=ADVANCED_FACE ( 'NONE', ( #12114 ), #18217, .F. ) ;
#12278=CARTESIAN_POINT ( 'NONE',  ( 6.626241948324199882, -16.73597674598852691, -32.00000000000000000 ) ) ;
#12284=DIRECTION ( 'NONE',  ( 0.000000000000000000, 0.000000000000000000, 1.000000000000000000 ) ) ;
#12286=EDGE_CURVE ( 'NONE', #9970, #18497, #11440, .T. ) ;
#12287=FACE_OUTER_BOUND ( 'NONE', #6102, .T. ) ;
#12288=AXIS2_PLACEMENT_3D ( 'NONE', #2404, #3909, #10031 ) ;
#12289=ORIENTED_EDGE ( 'NONE', *, *, #18222, .T. ) ;
#12294=CIRCLE ( 'NONE', #8462, 1.000000000000002442 ) ;
#12301=AXIS2_PLACEMENT_3D ( 'NONE', #14094, #15408, #18694 ) ;
#12309=LINE ( 'NONE', #12407, #6582 ) ;
#12311=DIRECTION ( 'NONE',  ( 1.000000000000000000, 0.000000000000000000, 0.000000000000000000 ) ) ;
#12313=CARTESIAN_POINT ( 'NONE',  ( 9.000000000000001776, 1.102182119232617911E-15, -30.00000000000000355 ) ) ;
#12317=LINE ( 'NONE', #16249, #18953 ) ;
#12322=EDGE_CURVE ( 'NONE', #12535, #4037, #10156, .T. ) ;
#12324=EDGE_LOOP ( 'NONE', ( #17095, #8117, #4821, #13364 ) ) ;
#12329=CIRCLE ( 'NONE', #2415, 1.000000000000002665 ) ;
#12333=CYLINDRICAL_SURFACE ( 'NONE', #11697, 9.000000000000000000 ) ;
#12336=VERTEX_POINT ( 'NONE', #15216 ) ;
#12343=CARTESIAN_POINT ( 'NONE',  ( 15.19790265903627358, 9.644882309621939598, 35.00000000000000000 ) ) ;
#12350=CIRCLE ( 'NONE', #11391, 1.000000000000000000 ) ;
#12351=EDGE_LOOP ( 'NONE', ( #18431, #18349, #12775, #3104 ) ) ;
#12355=ADVANCED_BREP_SHAPE_REPRESENTATION ( '', ( #15876, #16724 ), #7108 ) ;
#12357=DIRECTION ( 'NONE',  ( 1.000000000000000000, 0.000000000000000000, 0.000000000000000000 ) ) ;
#12360=( NAMED_UNIT ( * ) SI_UNIT ( $, .STERADIAN. ) SOLID_ANGLE_UNIT ( ) );
#12361=VERTEX_POINT ( 'NONE', #9308 ) ;
#12364=CARTESIAN_POINT ( 'NONE',  ( -13.86923836996420967, -11.47363181547641275, 32.00000000000000000 ) ) ;
#12371=ORIENTED_EDGE ( 'NONE', *, *, #8748, .T. ) ;
#12385=VERTEX_POINT ( 'NONE', #11003 ) ;
#12392=AXIS2_PLACEMENT_3D ( 'NONE', #4496, #16613, #18313 ) ;
#12395=VERTEX_POINT ( 'NONE', #6476 ) ;
#12405=ORIENTED_EDGE ( 'NONE', *, *, #3432, .F. ) ;
#12407=CARTESIAN_POINT ( 'NONE',  ( 11.58013454126452579, -14.56230589874905412, 32.00000000000000000 ) ) ;
#12408=CARTESIAN_POINT ( 'NONE',  ( 12.32184790671639618, 13.12143529358541016, -35.00000000000000000 ) ) ;
#12411=ORIENTED_EDGE ( 'NONE', *, *, #13701, .F. ) ;
#12418=DIRECTION ( 'NONE',  ( 0.000000000000000000, 0.000000000000000000, 1.000000000000000000 ) ) ;
#12430=ORIENTED_EDGE ( 'NONE', *, *, #11951, .T. ) ;
#12436=DIRECTION ( 'NONE',  ( 1.000000000000000000, 0.000000000000000000, 0.000000000000000000 ) ) ;
#12441=ORIENTED_EDGE ( 'NONE', *, *, #1149, .F. ) ;
#12461=ORIENTED_EDGE ( 'NONE', *, *, #8851, .F. ) ;
#12470=DIRECTION ( 'NONE',  ( 0.000000000000000000, 0.000000000000000000, -1.000000000000000000 ) ) ;
#12476=CIRCLE ( 'NONE', #19493, 1.000000000000004441 ) ;
#12490=EDGE_CURVE ( 'NONE', #12395, #1207, #15702, .T. ) ;
#12494=CARTESIAN_POINT ( 'NONE',  ( -18.68117051311639543, -3.372863662543042818, -32.00000000000000000 ) ) ;
#12496=CARTESIAN_POINT ( 'NONE',  ( 16.28688694438835327, -7.664027248171309203, 35.00000000000000000 ) ) ;
#12500=ORIENTED_EDGE ( 'NONE', *, *, #9981, .F. ) ;
#12502=CARTESIAN_POINT ( 'NONE',  ( -17.68117051311639898, -3.372863662543042818, -35.00000000000000000 ) ) ;
#12506=CIRCLE ( 'NONE', #11236, 1.000000000000000888 ) ;
#12512=CYLINDRICAL_SURFACE ( 'NONE', #4717, 1.000000000000004441 ) ;
#12528=CARTESIAN_POINT ( 'NONE',  ( 5.476417968967387750, 17.43449690031536292, -32.00000000000000000 ) ) ;
#12535=VERTEX_POINT ( 'NONE', #18896 ) ;
#12536=EDGE_CURVE ( 'NONE', #22, #4727, #11117, .T. ) ;
#12538=CARTESIAN_POINT ( 'NONE',  ( -13.86923836996420967, -11.47363181547641275, -32.00000000000000000 ) ) ;
#12540=CIRCLE ( 'NONE', #7393, 1.000000000000000888 ) ;
#12541=AXIS2_PLACEMENT_3D ( 'NONE', #6343, #9475, #1764 ) ;
#12547=VERTEX_POINT ( 'NONE', #799 ) ;
#12548=AXIS2_PLACEMENT_3D ( 'NONE', #16103, #3987, #13284 ) ;
#12553=DIRECTION ( 'NONE',  ( 1.000000000000000000, 0.000000000000000000, 0.000000000000000000 ) ) ;
#12556=DIRECTION ( 'NONE',  ( 1.000000000000000000, 0.000000000000000000, 0.000000000000000000 ) ) ;
#12557=DIRECTION ( 'NONE',  ( 1.000000000000000000, 0.000000000000000000, 0.000000000000000000 ) ) ;
#12562=AXIS2_PLACEMENT_3D ( 'NONE', #9755, #9856, #17543 ) ;
#12567=ORIENTED_EDGE ( 'NONE', *, *, #16075, .F. ) ;
#12579=DIRECTION ( 'NONE',  ( 1.000000000000000000, 0.000000000000000000, 0.000000000000000000 ) ) ;
#12580=VERTEX_POINT ( 'NONE', #14300 ) ;
#12587=CARTESIAN_POINT ( 'NONE',  ( 17.28688694438834972, -7.664027248171309203, 32.00000000000000000 ) ) ;
#12594=ORIENTED_EDGE ( 'NONE', *, *, #1125, .F. ) ;
#12597=ADVANCED_FACE ( 'NONE', ( #6778 ), #601, .F. ) ;
#12600=CIRCLE ( 'NONE', #13548, 1.000000000000000888 ) ;
#12606=CARTESIAN_POINT ( 'NONE',  ( 17.11901729331276556, 5.562305898749055011, 32.00000000000000000 ) ) ;
#12607=EDGE_CURVE ( 'NONE', #4727, #22, #18467, .T. ) ;
#12608=CARTESIAN_POINT ( 'NONE',  ( -7.671566133830872047, 15.77352024078954429, 32.00000000000000000 ) ) ;
#12609=ORIENTED_EDGE ( 'NONE', *, *, #10628, .T. ) ;
#12611=VECTOR ( 'NONE', #45, 1000.000000000000000 ) ;
#12614=DIRECTION ( 'NONE',  ( 0.000000000000000000, 0.000000000000000000, -1.000000000000000000 ) ) ;
#12621=VERTEX_POINT ( 'NONE', #2771 ) ;
#12631=DIRECTION ( 'NONE',  ( 0.000000000000000000, 0.000000000000000000, 1.000000000000000000 ) ) ;
#12633=EDGE_CURVE ( 'NONE', #3138, #13831, #5874, .T. ) ;
#12634=DIRECTION ( 'NONE',  ( 1.000000000000000000, 0.000000000000000000, 0.000000000000000000 ) ) ;
#12641=AXIS2_PLACEMENT_3D ( 'NONE', #12178, #13878, #68 ) ;
#12646=EDGE_LOOP ( 'NONE', ( #3167, #17649 ) ) ;
#12648=ADVANCED_FACE ( 'NONE', ( #1183 ), #18194, .F. ) ;
#12649=CARTESIAN_POINT ( 'NONE',  ( -10.58013454126452224, -14.56230589874905235, -35.00000000000000000 ) ) ;
#12663=ORIENTED_EDGE ( 'NONE', *, *, #18962, .F. ) ;
#12667=EDGE_CURVE ( 'NONE', #9386, #3914, #12719, .T. ) ;
#12670=CIRCLE ( 'NONE', #4036, 9.000000000000001776 ) ;
#12672=ORIENTED_EDGE ( 'NONE', *, *, #18017, .F. ) ;
#12674=LINE ( 'NONE', #4866, #8716 ) ;
#12675=FACE_BOUND ( 'NONE', #8165, .T. ) ;
#12676=ORIENTED_EDGE ( 'NONE', *, *, #12165, .T. ) ;
#12690=VERTEX_POINT ( 'NONE', #1482 ) ;
#12692=ADVANCED_FACE ( 'NONE', ( #15089 ), #4477, .F. ) ;
#12695=CARTESIAN_POINT ( 'NONE',  ( -8.671566133830875600, 15.77352024078954429, -35.00000000000000000 ) ) ;
#12698=ORIENTED_EDGE ( 'NONE', *, *, #4560, .F. ) ;
#12704=AXIS2_PLACEMENT_3D ( 'NONE', #18924, #11429, #5316 ) ;
#12713=ORIENTED_EDGE ( 'NONE', *, *, #4521, .T. ) ;
#12719=CIRCLE ( 'NONE', #894, 22.00000000000000355 ) ;
#12720=AXIS2_PLACEMENT_3D ( 'NONE', #13617, #13814, #18031 ) ;
#12722=CYLINDRICAL_SURFACE ( 'NONE', #14509, 1.000000000000002665 ) ;
#12725=PRESENTATION_STYLE_ASSIGNMENT (( #7640 ) ) ;
#12734=EDGE_CURVE ( 'NONE', #12395, #7772, #4731, .T. ) ;
#12739=ORIENTED_EDGE ( 'NONE', *, *, #14959, .T. ) ;
#12740=FACE_BOUND ( 'NONE', #8078, .T. ) ;
#12744=EDGE_CURVE ( 'NONE', #8623, #12225, #5987, .T. ) ;
#12745=CARTESIAN_POINT ( 'NONE',  ( -6.626241948324210540, -16.73597674598852336, -32.00000000000000000 ) ) ;
#12749=CARTESIAN_POINT ( 'NONE',  ( 7.626241948324204323, -16.73597674598852691, -35.00000000000000000 ) ) ;
#12755=ORIENTED_EDGE ( 'NONE', *, *, #14677, .F. ) ;
#12760=VERTEX_POINT ( 'NONE', #5575 ) ;
#12775=ORIENTED_EDGE ( 'NONE', *, *, #6616, .T. ) ;
#12779=VERTEX_POINT ( 'NONE', #13383 ) ;
#12780=ORIENTED_EDGE ( 'NONE', *, *, #18271, .T. ) ;
#12782=AXIS2_PLACEMENT_3D ( 'NONE', #430, #1731, #12436 ) ;
#12792=AXIS2_PLACEMENT_3D ( 'NONE', #3378, #10691, #13785 ) ;
#12798=DIRECTION ( 'NONE',  ( 0.000000000000000000, 0.000000000000000000, -1.000000000000000000 ) ) ;
#12802=CARTESIAN_POINT ( 'NONE',  ( 17.96448111170888851, 1.130229351527639148, -32.00000000000000000 ) ) ;
#12805=CARTESIAN_POINT ( 'NONE',  ( -1.000000000000001998, 18.00000000000000355, 35.00000000000000000 ) ) ;
#12809=CARTESIAN_POINT ( 'NONE',  ( -18.11901729331277267, 5.562305898749051458, -32.00000000000000000 ) ) ;
#12820=VERTEX_POINT ( 'NONE', #1774 ) ;
#12821=VECTOR ( 'NONE', #3035, 1000.000000000000000 ) ;
#12827=CYLINDRICAL_SURFACE ( 'NONE', #3436, 1.000000000000000888 ) ;
#12831=DIRECTION ( 'NONE',  ( 0.000000000000000000, 0.000000000000000000, 1.000000000000000000 ) ) ;
#12832=DIRECTION ( 'NONE',  ( 1.000000000000000000, 0.000000000000000000, 0.000000000000000000 ) ) ;
#12835=FACE_OUTER_BOUND ( 'NONE', #17191, .T. ) ;
#12839=AXIS2_PLACEMENT_3D ( 'NONE', #7347, #2861, #13573 ) ;
#12843=FACE_OUTER_BOUND ( 'NONE', #9265, .T. ) ;
#12865=ORIENTED_EDGE ( 'NONE', *, *, #4682, .T. ) ;
#12883=CYLINDRICAL_SURFACE ( 'NONE', #8174, 1.000000000000004441 ) ;
#12888=EDGE_LOOP ( 'NONE', ( #6777, #17122 ) ) ;
#12897=CARTESIAN_POINT ( 'NONE',  ( 8.671566133830875600, 15.77352024078954784, 35.00000000000000000 ) ) ;
#12899=LINE ( 'NONE', #14695, #8695 ) ;
#12904=CARTESIAN_POINT ( 'NONE',  ( -18.11901729331277267, 5.562305898749051458, -35.00000000000000000 ) ) ;
#12913=ORIENTED_EDGE ( 'NONE', *, *, #2669, .F. ) ;
#12928=EDGE_LOOP ( 'NONE', ( #13969, #18203, #10915, #17348 ) ) ;
#12933=CIRCLE ( 'NONE', #7479, 1.000000000000000888 ) ;
#12935=CARTESIAN_POINT ( 'NONE',  ( -9.000000000000000000, 1.102182119232617714E-15, 35.00000000000000000 ) ) ;
#12937=EDGE_LOOP ( 'NONE', ( #17499, #15768, #5559, #19145 ) ) ;
#12938=CARTESIAN_POINT ( 'NONE',  ( 0.000000000000000000, 0.000000000000000000, 32.00000000000000000 ) ) ;
#12939=EDGE_CURVE ( 'NONE', #8859, #18804, #16577, .T. ) ;
#12946=CYLINDRICAL_SURFACE ( 'NONE', #12188, 1.000000000000002887 ) ;
#12949=CYLINDRICAL_SURFACE ( 'NONE', #2360, 0.9999999999999974465 ) ;
#12963=CARTESIAN_POINT ( 'NONE',  ( -17.68117051311639898, -3.372863662543042818, 35.00000000000000000 ) ) ;
#12964=DIRECTION ( 'NONE',  ( 0.000000000000000000, 0.000000000000000000, 1.000000000000000000 ) ) ;
#12970=AXIS2_PLACEMENT_3D ( 'NONE', #4562, #1466, #7446 ) ;
#12973=DIRECTION ( 'NONE',  ( 1.000000000000000000, 0.000000000000000000, 0.000000000000000000 ) ) ;
#12984=CARTESIAN_POINT ( 'NONE',  ( -12.32184790671639085, 13.12143529358541549, -32.00000000000000000 ) ) ;
#12993=CARTESIAN_POINT ( 'NONE',  ( 0.000000000000000000, 0.000000000000000000, 29.00000000000000355 ) ) ;
#12996=DIRECTION ( 'NONE',  ( 0.000000000000000000, 0.000000000000000000, 1.000000000000000000 ) ) ;
#13001=EDGE_CURVE ( 'NONE', #3237, #18640, #18976, .T. ) ;
#13012=VERTEX_POINT ( 'NONE', #14280 ) ;
#13017=CARTESIAN_POINT ( 'NONE',  ( -22.00000000000000355, 2.694222958124177204E-15, 32.00000000000000000 ) ) ;
#13027=EDGE_LOOP ( 'NONE', ( #7329, #2315 ) ) ;
#13034=ORIENTED_EDGE ( 'NONE', *, *, #8974, .F. ) ;
#13035=FACE_BOUND ( 'NONE', #4994, .T. ) ;
#13042=ORIENTED_EDGE ( 'NONE', *, *, #10069, .F. ) ;
#13043=LINE ( 'NONE', #16046, #11991 ) ;
#13045=FACE_BOUND ( 'NONE', #15287, .T. ) ;
#13048=AXIS2_PLACEMENT_3D ( 'NONE', #5385, #5187, #14404 ) ;
#13049=VERTEX_POINT ( 'NONE', #17381 ) ;
#13057=FACE_OUTER_BOUND ( 'NONE', #11248, .T. ) ;
#13059=EDGE_CURVE ( 'NONE', #15888, #16011, #6967, .T. ) ;
#13063=CIRCLE ( 'NONE', #15937, 1.000000000000002665 ) ;
#13070=CARTESIAN_POINT ( 'NONE',  ( -2.255998204157477538, -17.85806462366060288, 35.00000000000000000 ) ) ;
#13072=ORIENTED_EDGE ( 'NONE', *, *, #15007, .T. ) ;
#13074=DIRECTION ( 'NONE',  ( 0.000000000000000000, 0.000000000000000000, 1.000000000000000000 ) ) ;
#13078=DIRECTION ( 'NONE',  ( -0.000000000000000000, -0.000000000000000000, 1.000000000000000000 ) ) ;
#13080=DIRECTION ( 'NONE',  ( 0.000000000000000000, 0.000000000000000000, 1.000000000000000000 ) ) ;
#13086=ADVANCED_FACE ( 'NONE', ( #13270 ), #2651, .F. ) ;
#13088=EDGE_CURVE ( 'NONE', #5753, #11765, #13063, .T. ) ;
#13094=CARTESIAN_POINT ( 'NONE',  ( -10.58013454126452224, -14.56230589874905235, 32.00000000000000000 ) ) ;
#13095=EDGE_CURVE ( 'NONE', #12361, #14452, #17535, .T. ) ;
#13101=ORIENTED_EDGE ( 'NONE', *, *, #9015, .T. ) ;
#13103=DIRECTION ( 'NONE',  ( 0.000000000000000000, 0.000000000000000000, 1.000000000000000000 ) ) ;
#13104=AXIS2_PLACEMENT_3D ( 'NONE', #11032, #6312, #9744 ) ;
#13106=DIRECTION ( 'NONE',  ( 0.000000000000000000, 0.000000000000000000, -1.000000000000000000 ) ) ;
#13115=EDGE_CURVE ( 'NONE', #7654, #1041, #10507, .T. ) ;
#13116=CARTESIAN_POINT ( 'NONE',  ( 0.000000000000000000, 0.000000000000000000, 29.00000000000000355 ) ) ;
#13118=ORIENTED_EDGE ( 'NONE', *, *, #8943, .F. ) ;
#13122=CIRCLE ( 'NONE', #16954, 1.000000000000004441 ) ;
#13124=DIRECTION ( 'NONE',  ( -1.000000000000000000, 0.000000000000000000, 0.000000000000000000 ) ) ;
#13129=FACE_BOUND ( 'NONE', #440, .T. ) ;
#13130=CARTESIAN_POINT ( 'NONE',  ( 16.96448111170888851, 1.130229351527639148, -35.00000000000000000 ) ) ;
#13131=ORIENTED_EDGE ( 'NONE', *, *, #13538, .T. ) ;
#13135=EDGE_CURVE ( 'NONE', #13172, #7172, #9224, .T. ) ;
#13140=DIRECTION ( 'NONE',  ( 1.000000000000000000, 0.000000000000000000, -0.000000000000000000 ) ) ;
#13146=CARTESIAN_POINT ( 'NONE',  ( 11.32184790671639263, 13.12143529358541016, -32.00000000000000000 ) ) ;
#13149=CARTESIAN_POINT ( 'NONE',  ( 13.86923836996420789, -11.47363181547641453, -32.00000000000000000 ) ) ;
#13150=CIRCLE ( 'NONE', #2591, 1.000000000000002665 ) ;
#13151=CIRCLE ( 'NONE', #9648, 14.00000000000000178 ) ;
#13155=APPLICATION_CONTEXT ( 'automotive_design' ) ;
#13157=ADVANCED_FACE ( 'NONE', ( #4263 ), #1261, .F. ) ;
#13161=AXIS2_PLACEMENT_3D ( 'NONE', #4883, #7872, #4587 ) ;
#13162=CARTESIAN_POINT ( 'NONE',  ( -16.19790265903627713, 9.644882309621941374, -35.00000000000000000 ) ) ;
#13171=ORIENTED_EDGE ( 'NONE', *, *, #13847, .F. ) ;
#13172=VERTEX_POINT ( 'NONE', #962 ) ;
#13173=DIRECTION ( 'NONE',  ( 0.000000000000000000, 0.000000000000000000, 1.000000000000000000 ) ) ;
#13174=EDGE_CURVE ( 'NONE', #7627, #6695, #14018, .T. ) ;
#13182=CYLINDRICAL_SURFACE ( 'NONE', #18416, 1.000000000000000888 ) ;
#13185=AXIS2_PLACEMENT_3D ( 'NONE', #17673, #8371, #14673 ) ;
#13187=EDGE_CURVE ( 'NONE', #11765, #17321, #7141, .T. ) ;
#13211=EDGE_CURVE ( 'NONE', #16953, #14278, #18792, .T. ) ;
#13212=EDGE_CURVE ( 'NONE', #4121, #14720, #18178, .T. ) ;
#13220=CARTESIAN_POINT ( 'NONE',  ( -15.19790265903627180, 9.644882309621941374, -32.00000000000000000 ) ) ;
#13233=EDGE_LOOP ( 'NONE', ( #5099, #2438 ) ) ;
#13234=AXIS2_PLACEMENT_3D ( 'NONE', #17057, #14146, #12357 ) ;
#13246=EDGE_LOOP ( 'NONE', ( #7899, #261 ) ) ;
#13248=ORIENTED_EDGE ( 'NONE', *, *, #16075, .T. ) ;
#13249=DIRECTION ( 'NONE',  ( 0.000000000000000000, 0.000000000000000000, -1.000000000000000000 ) ) ;
#13254=DIRECTION ( 'NONE',  ( 1.000000000000000000, 0.000000000000000000, 0.000000000000000000 ) ) ;
#13270=FACE_OUTER_BOUND ( 'NONE', #9326, .T. ) ;
#13272=VERTEX_POINT ( 'NONE', #6047 ) ;
#13273=VECTOR ( 'NONE', #5173, 1000.000000000000000 ) ;
#13274=DIRECTION ( 'NONE',  ( -0.000000000000000000, -0.000000000000000000, 1.000000000000000000 ) ) ;
#13276=DIRECTION ( 'NONE',  ( -0.000000000000000000, -0.000000000000000000, 1.000000000000000000 ) ) ;
#13279=LINE ( 'NONE', #4274, #9123 ) ;
#13280=DIRECTION ( 'NONE',  ( 1.000000000000000000, 0.000000000000000000, 0.000000000000000000 ) ) ;
#13284=DIRECTION ( 'NONE',  ( 1.000000000000000000, 0.000000000000000000, 0.000000000000000000 ) ) ;
#13287=DIRECTION ( 'NONE',  ( -0.000000000000000000, -0.000000000000000000, 1.000000000000000000 ) ) ;
#13292=EDGE_CURVE ( 'NONE', #12779, #16239, #18481, .T. ) ;
#13294=CYLINDRICAL_SURFACE ( 'NONE', #16680, 1.000000000000002665 ) ;
#13300=CARTESIAN_POINT ( 'NONE',  ( -16.96448111170888851, 1.130229351527647808, -32.00000000000000000 ) ) ;
#13307=ORIENTED_EDGE ( 'NONE', *, *, #15225, .F. ) ;
#13310=ORIENTED_EDGE ( 'NONE', *, *, #12607, .F. ) ;
#13311=CARTESIAN_POINT ( 'NONE',  ( -10.58013454126452224, -14.56230589874905235, -32.00000000000000000 ) ) ;
#13314=FACE_OUTER_BOUND ( 'NONE', #13626, .T. ) ;
#13318=CYLINDRICAL_SURFACE ( 'NONE', #2592, 1.000000000000002665 ) ;
#13319=DIRECTION ( 'NONE',  ( 0.000000000000000000, 0.000000000000000000, -1.000000000000000000 ) ) ;
#13329=DIRECTION ( 'NONE',  ( 0.000000000000000000, 0.000000000000000000, 1.000000000000000000 ) ) ;
#13334=CARTESIAN_POINT ( 'NONE',  ( -2.255998204157477538, -17.85806462366060288, 32.00000000000000000 ) ) ;
#13341=AXIS2_PLACEMENT_3D ( 'NONE', #17329, #128, #12634 ) ;
#13343=CIRCLE ( 'NONE', #19083, 1.000000000000000888 ) ;
#13344=ORIENTED_EDGE ( 'NONE', *, *, #11308, .F. ) ;
#13346=CARTESIAN_POINT ( 'NONE',  ( 13.86923836996420789, -11.47363181547641453, 32.00000000000000000 ) ) ;
#13355=CYLINDRICAL_SURFACE ( 'NONE', #18984, 1.000000000000000888 ) ;
#13356=EDGE_CURVE ( 'NONE', #1041, #7654, #18188, .T. ) ;
#13358=CYLINDRICAL_SURFACE ( 'NONE', #9280, 1.000000000000004441 ) ;
#13361=ORIENTED_EDGE ( 'NONE', *, *, #3354, .T. ) ;
#13362=DIRECTION ( 'NONE',  ( 1.000000000000000000, 0.000000000000000000, 0.000000000000000000 ) ) ;
#13364=ORIENTED_EDGE ( 'NONE', *, *, #16965, .F. ) ;
#13368=CARTESIAN_POINT ( 'NONE',  ( -3.255998204157480203, -17.85806462366060288, 32.00000000000000000 ) ) ;
#13377=EDGE_CURVE ( 'NONE', #4037, #12535, #8582, .T. ) ;
#13378=VECTOR ( 'NONE', #12614, 1000.000000000000000 ) ;
#13383=CARTESIAN_POINT ( 'NONE',  ( -15.28688694438835505, -7.664027248171298545, 32.00000000000000000 ) ) ;
#13384=CARTESIAN_POINT ( 'NONE',  ( -17.96448111170888851, 1.130229351527647585, -32.00000000000000000 ) ) ;
#13390=EDGE_LOOP ( 'NONE', ( #13034, #8293 ) ) ;
#13402=DIRECTION ( 'NONE',  ( 1.000000000000000000, 0.000000000000000000, 0.000000000000000000 ) ) ;
#13411=EDGE_CURVE ( 'NONE', #4459, #17830, #14984, .T. ) ;
#13413=AXIS2_PLACEMENT_3D ( 'NONE', #4626, #6502, #7819 ) ;
#13414=ORIENTED_EDGE ( 'NONE', *, *, #3586, .F. ) ;
#13416=EDGE_LOOP ( 'NONE', ( #17605, #16558, #9364, #17479 ) ) ;
#13425=FACE_BOUND ( 'NONE', #15314, .T. ) ;
#13427=EDGE_LOOP ( 'NONE', ( #12441, #10567 ) ) ;
#13436=CARTESIAN_POINT ( 'NONE',  ( 6.626241948324199882, -16.73597674598852691, 32.00000000000000000 ) ) ;
#13437=ORIENTED_EDGE ( 'NONE', *, *, #17088, .F. ) ;
#13450=AXIS2_PLACEMENT_3D ( 'NONE', #14858, #9801, #2178 ) ;
#13462=DIRECTION ( 'NONE',  ( -0.000000000000000000, -0.000000000000000000, 1.000000000000000000 ) ) ;
#13463=SHAPE_REPRESENTATION ( 'Outer Wheel Hub Shell', ( #16724 ), #7108 ) ;
#13473=FACE_OUTER_BOUND ( 'NONE', #6995, .T. ) ;
#13476=DIRECTION ( 'NONE',  ( 0.000000000000000000, 0.000000000000000000, 1.000000000000000000 ) ) ;
#13481=CARTESIAN_POINT ( 'NONE',  ( -3.476417968967383754, 17.43449690031536292, 35.00000000000000000 ) ) ;
#13484=EDGE_CURVE ( 'NONE', #12580, #2419, #2532, .T. ) ;
#13490=CIRCLE ( 'NONE', #65, 1.000000000000004441 ) ;
#13506=DIRECTION ( 'NONE',  ( 0.000000000000000000, 0.000000000000000000, 1.000000000000000000 ) ) ;
#13510=CARTESIAN_POINT ( 'NONE',  ( -18.96448111170889206, 1.130229351527647808, 35.00000000000000000 ) ) ;
#13515=DIRECTION ( 'NONE',  ( 1.000000000000000000, 0.000000000000000000, 0.000000000000000000 ) ) ;
#13516=ORIENTED_EDGE ( 'NONE', *, *, #9552, .F. ) ;
#13526=APPLICATION_CONTEXT ( 'automotive_design' ) ;
#13530=ORIENTED_EDGE ( 'NONE', *, *, #4850, .T. ) ;
#13532=EDGE_LOOP ( 'NONE', ( #9965, #18162 ) ) ;
#13536=AXIS2_PLACEMENT_3D ( 'NONE', #11904, #2888, #9003 ) ;
#13537=DIRECTION ( 'NONE',  ( -1.000000000000000000, 0.000000000000000000, 0.000000000000000000 ) ) ;
#13538=EDGE_CURVE ( 'NONE', #344, #12048, #12104, .T. ) ;
#13543=FACE_OUTER_BOUND ( 'NONE', #14260, .T. ) ;
#13547=VERTEX_POINT ( 'NONE', #2727 ) ;
#13548=AXIS2_PLACEMENT_3D ( 'NONE', #18496, #17005, #9405 ) ;
#13549=DIRECTION ( 'NONE',  ( -0.000000000000000000, -0.000000000000000000, -1.000000000000000000 ) ) ;
#13557=AXIS2_PLACEMENT_3D ( 'NONE', #3840, #19143, #10058 ) ;
#13561=CARTESIAN_POINT ( 'NONE',  ( -4.476417968967385974, 17.43449690031536292, -35.00000000000000000 ) ) ;
#13564=ORIENTED_EDGE ( 'NONE', *, *, #18821, .T. ) ;
#13572=DIRECTION ( 'NONE',  ( 1.000000000000000000, 0.000000000000000000, 0.000000000000000000 ) ) ;
#13573=DIRECTION ( 'NONE',  ( -1.000000000000000000, 0.000000000000000000, 0.000000000000000000 ) ) ;
#13581=CARTESIAN_POINT ( 'NONE',  ( 12.32184790671639618, 13.12143529358541016, -32.00000000000000000 ) ) ;
#13583=EDGE_CURVE ( 'NONE', #11765, #5753, #2199, .T. ) ;
#13584=CARTESIAN_POINT ( 'NONE',  ( 0.000000000000000000, 0.000000000000000000, -35.00000000000000000 ) ) ;
#13586=FACE_BOUND ( 'NONE', #228, .T. ) ;
#13589=DIRECTION ( 'NONE',  ( -1.000000000000000000, 0.000000000000000000, 0.000000000000000000 ) ) ;
#13592=ORIENTED_EDGE ( 'NONE', *, *, #10073, .T. ) ;
#13593=CARTESIAN_POINT ( 'NONE',  ( 14.19790265903627180, 9.644882309621939598, 32.00000000000000000 ) ) ;
#13596=ORIENTED_EDGE ( 'NONE', *, *, #2197, .T. ) ;
#13601=CARTESIAN_POINT ( 'NONE',  ( 2.255998204157473097, -17.85806462366060288, -35.00000000000000000 ) ) ;
#13617=CARTESIAN_POINT ( 'NONE',  ( -17.68117051311639898, -3.372863662543042818, -32.00000000000000000 ) ) ;
#13622=ORIENTED_EDGE ( 'NONE', *, *, #84, .F. ) ;
#13623=EDGE_CURVE ( 'NONE', #6438, #4912, #14029, .T. ) ;
#13626=EDGE_LOOP ( 'NONE', ( #8240, #4968, #9089, #1935 ) ) ;
#13632=ORIENTED_EDGE ( 'NONE', *, *, #5649, .F. ) ;
#13636=ORIENTED_EDGE ( 'NONE', *, *, #6299, .T. ) ;
#13637=CARTESIAN_POINT ( 'NONE',  ( -6.626241948324210540, -16.73597674598852336, -35.00000000000000000 ) ) ;
#13644=LINE ( 'NONE', #7319, #7097 ) ;
#13645=CIRCLE ( 'NONE', #11725, 1.000000000000002442 ) ;
#13646=AXIS2_PLACEMENT_3D ( 'NONE', #12538, #11033, #18830 ) ;
#13648=ORIENTED_EDGE ( 'NONE', *, *, #3779, .F. ) ;
#13665=ORIENTED_EDGE ( 'NONE', *, *, #19384, .T. ) ;
#13666=VERTEX_POINT ( 'NONE', #10643 ) ;
#13672=EDGE_LOOP ( 'NONE', ( #6835, #6261 ) ) ;
#13674=AXIS2_PLACEMENT_3D ( 'NONE', #5966, #19383, #12090 ) ;
#13676=VECTOR ( 'NONE', #6385, 1000.000000000000000 ) ;
#13688=FACE_BOUND ( 'NONE', #16480, .T. ) ;
#13690=CARTESIAN_POINT ( 'NONE',  ( 12.32184790671639618, 13.12143529358541016, -32.00000000000000000 ) ) ;
#13696=CARTESIAN_POINT ( 'NONE',  ( 14.19790265903627180, 9.644882309621939598, -35.00000000000000000 ) ) ;
#13697=ADVANCED_FACE ( 'NONE', ( #15247, #18146 ), #14104, .F. ) ;
#13701=EDGE_CURVE ( 'NONE', #19705, #14268, #3501, .T. ) ;
#13702=EDGE_LOOP ( 'NONE', ( #4640, #14613 ) ) ;
#13709=EDGE_CURVE ( 'NONE', #12361, #10647, #13738, .T. ) ;
#13712=LINE ( 'NONE', #8913, #1930 ) ;
#13722=DIRECTION ( 'NONE',  ( 0.000000000000000000, 0.000000000000000000, 1.000000000000000000 ) ) ;
#13731=ORIENTED_EDGE ( 'NONE', *, *, #7547, .F. ) ;
#13738=LINE ( 'NONE', #18700, #6983 ) ;
#13757=CARTESIAN_POINT ( 'NONE',  ( 11.58013454126452579, -14.56230589874905412, -32.00000000000000000 ) ) ;
#13763=DIRECTION ( 'NONE',  ( 1.000000000000000000, 0.000000000000000000, 0.000000000000000000 ) ) ;
#13766=EDGE_CURVE ( 'NONE', #6991, #12580, #19137, .T. ) ;
#13767=ORIENTED_EDGE ( 'NONE', *, *, #1813, .T. ) ;
#13768=CARTESIAN_POINT ( 'NONE',  ( -17.68117051311639898, -3.372863662543042818, 32.00000000000000000 ) ) ;
#13773=DIRECTION ( 'NONE',  ( 0.000000000000000000, 0.000000000000000000, -1.000000000000000000 ) ) ;
#13778=EDGE_CURVE ( 'NONE', #6546, #12760, #17506, .T. ) ;
#13785=DIRECTION ( 'NONE',  ( 1.000000000000000000, 0.000000000000000000, 0.000000000000000000 ) ) ;
#13786=CYLINDRICAL_SURFACE ( 'NONE', #3259, 1.000000000000000888 ) ;
#13788=LINE ( 'NONE', #5679, #2810 ) ;
#13799=VERTEX_POINT ( 'NONE', #12805 ) ;
#13804=DIRECTION ( 'NONE',  ( 0.000000000000000000, 0.000000000000000000, -1.000000000000000000 ) ) ;
#13805=EDGE_LOOP ( 'NONE', ( #15300, #10766, #13828, #12371 ) ) ;
#13814=DIRECTION ( 'NONE',  ( 0.000000000000000000, 0.000000000000000000, -1.000000000000000000 ) ) ;
#13818=CIRCLE ( 'NONE', #12224, 1.000000000000000888 ) ;
#13824=VECTOR ( 'NONE', #14560, 1000.000000000000000 ) ;
#13828=ORIENTED_EDGE ( 'NONE', *, *, #11529, .T. ) ;
#13829=CYLINDRICAL_SURFACE ( 'NONE', #9802, 1.000000000000000888 ) ;
#13831=VERTEX_POINT ( 'NONE', #357 ) ;
#13837=CARTESIAN_POINT ( 'NONE',  ( -17.11901729331276911, 5.562305898749051458, 32.00000000000000000 ) ) ;
#13847=EDGE_CURVE ( 'NONE', #5711, #14278, #2157, .T. ) ;
#13849=EDGE_LOOP ( 'NONE', ( #15495, #1673 ) ) ;
#13856=ORIENTED_EDGE ( 'NONE', *, *, #9669, .T. ) ;
#13869=EDGE_CURVE ( 'NONE', #4563, #7726, #16924, .T. ) ;
#13874=AXIS2_PLACEMENT_3D ( 'NONE', #937, #7016, #13140 ) ;
#13878=DIRECTION ( 'NONE',  ( -0.000000000000000000, -0.000000000000000000, 1.000000000000000000 ) ) ;
#13898=AXIS2_PLACEMENT_3D ( 'NONE', #3192, #12110, #2995 ) ;
#13900=DIRECTION ( 'NONE',  ( 1.000000000000000000, 0.000000000000000000, 0.000000000000000000 ) ) ;
#13903=AXIS2_PLACEMENT_3D ( 'NONE', #10406, #5885, #14807 ) ;
#13907=VERTEX_POINT ( 'NONE', #14269 ) ;
#13921=ORIENTED_EDGE ( 'NONE', *, *, #14344, .T. ) ;
#13929=EDGE_LOOP ( 'NONE', ( #17749, #13767 ) ) ;
#13932=DIRECTION ( 'NONE',  ( -0.000000000000000000, -0.000000000000000000, 1.000000000000000000 ) ) ;
#13933=AXIS2_PLACEMENT_3D ( 'NONE', #19449, #8857, #5738 ) ;
#13935=DIRECTION ( 'NONE',  ( -0.000000000000000000, -0.000000000000000000, 1.000000000000000000 ) ) ;
#13936=ADVANCED_FACE ( 'NONE', ( #3556 ), #9680, .F. ) ;
#13938=CARTESIAN_POINT ( 'NONE',  ( 2.255998204157473097, -17.85806462366060288, 35.00000000000000000 ) ) ;
#13943=CARTESIAN_POINT ( 'NONE',  ( -17.96448111170888851, 1.130229351527647585, 32.00000000000000000 ) ) ;
#13948=EDGE_CURVE ( 'NONE', #13547, #2023, #15000, .T. ) ;
#13954=DIRECTION ( 'NONE',  ( -0.000000000000000000, -0.000000000000000000, -1.000000000000000000 ) ) ;
#13955=EDGE_CURVE ( 'NONE', #18092, #3037, #305, .T. ) ;
#13961=ORIENTED_EDGE ( 'NONE', *, *, #9048, .F. ) ;
#13963=DIRECTION ( 'NONE',  ( 1.000000000000000000, 0.000000000000000000, 0.000000000000000000 ) ) ;
#13967=CARTESIAN_POINT ( 'NONE',  ( -15.19790265903627180, 9.644882309621941374, 35.00000000000000000 ) ) ;
#13969=ORIENTED_EDGE ( 'NONE', *, *, #18687, .F. ) ;
#13975=CARTESIAN_POINT ( 'NONE',  ( -2.255998204157477538, -17.85806462366060288, -32.00000000000000000 ) ) ;
#13986=CARTESIAN_POINT ( 'NONE',  ( 16.19790265903627358, 9.644882309621939598, -35.00000000000000000 ) ) ;
#13987=AXIS2_PLACEMENT_3D ( 'NONE', #7822, #13932, #17037 ) ;
#13990=VERTEX_POINT ( 'NONE', #770 ) ;
#13998=EDGE_CURVE ( 'NONE', #12385, #8529, #14861, .T. ) ;
#13999=DIRECTION ( 'NONE',  ( -1.000000000000000000, 0.000000000000000000, 0.000000000000000000 ) ) ;
#14003=DIRECTION ( 'NONE',  ( 0.000000000000000000, 0.000000000000000000, 1.000000000000000000 ) ) ;
#14014=ORIENTED_EDGE ( 'NONE', *, *, #18131, .F. ) ;
#14017=DIRECTION ( 'NONE',  ( 0.000000000000000000, 0.000000000000000000, -1.000000000000000000 ) ) ;
#14018=CIRCLE ( 'NONE', #7275, 1.000000000000002665 ) ;
#14028=ORIENTED_EDGE ( 'NONE', *, *, #5596, .F. ) ;
#14029=CIRCLE ( 'NONE', #9236, 1.000000000000002665 ) ;
#14031=ORIENTED_EDGE ( 'NONE', *, *, #19071, .F. ) ;
#14045=AXIS2_PLACEMENT_3D ( 'NONE', #13561, #1459, #14965 ) ;
#14047=VERTEX_POINT ( 'NONE', #13162 ) ;
#14052=FACE_OUTER_BOUND ( 'NONE', #14473, .T. ) ;
#14055=DIRECTION ( 'NONE',  ( 0.000000000000000000, 0.000000000000000000, 1.000000000000000000 ) ) ;
#14065=DIRECTION ( 'NONE',  ( 0.000000000000000000, 0.000000000000000000, -1.000000000000000000 ) ) ;
#14066=CARTESIAN_POINT ( 'NONE',  ( 0.000000000000000000, 0.000000000000000000, -32.00000000000000000 ) ) ;
#14069=CARTESIAN_POINT ( 'NONE',  ( 18.11901729331276911, 5.562305898749055011, -32.00000000000000000 ) ) ;
#14091=EDGE_LOOP ( 'NONE', ( #9201, #15976, #8759, #705 ) ) ;
#14094=CARTESIAN_POINT ( 'NONE',  ( 13.86923836996420789, -11.47363181547641453, 32.00000000000000000 ) ) ;
#14104=PLANE ( 'NONE',  #14345 ) ;
#14108=EDGE_CURVE ( 'NONE', #6632, #15965, #1571, .T. ) ;
#14121=CIRCLE ( 'NONE', #11567, 1.000000000000002665 ) ;
#14131=DIRECTION ( 'NONE',  ( 0.000000000000000000, 0.000000000000000000, 1.000000000000000000 ) ) ;
#14132=VECTOR ( 'NONE', #1071, 1000.000000000000000 ) ;
#14137=FACE_OUTER_BOUND ( 'NONE', #2822, .T. ) ;
#14139=EDGE_LOOP ( 'NONE', ( #15927, #18479 ) ) ;
#14141=DIRECTION ( 'NONE',  ( -0.000000000000000000, -0.000000000000000000, 1.000000000000000000 ) ) ;
#14142=CARTESIAN_POINT ( 'NONE',  ( -17.96448111170888851, 1.130229351527647585, 35.00000000000000000 ) ) ;
#14146=DIRECTION ( 'NONE',  ( 0.000000000000000000, 0.000000000000000000, 1.000000000000000000 ) ) ;
#14157=ORIENTED_EDGE ( 'NONE', *, *, #10872, .F. ) ;
#14159=DIRECTION ( 'NONE',  ( 0.000000000000000000, 0.000000000000000000, -1.000000000000000000 ) ) ;
#14171=EDGE_LOOP ( 'NONE', ( #3505, #5160, #13636, #3798 ) ) ;
#14178=ADVANCED_FACE ( 'NONE', ( #1936 ), #18449, .F. ) ;
#14185=DIRECTION ( 'NONE',  ( 0.000000000000000000, 0.000000000000000000, -1.000000000000000000 ) ) ;
#14186=CIRCLE ( 'NONE', #7137, 22.00000000000000355 ) ;
#14195=EDGE_LOOP ( 'NONE', ( #13731, #15066, #9591, #1326 ) ) ;
#14196=DIRECTION ( 'NONE',  ( 0.000000000000000000, 0.000000000000000000, 1.000000000000000000 ) ) ;
#14202=AXIS2_PLACEMENT_3D ( 'NONE', #11272, #11070, #11173 ) ;
#14206=CARTESIAN_POINT ( 'NONE',  ( 22.00000000000000355, 2.694222958124177204E-15, -35.00000000000000000 ) ) ;
#14209=ADVANCED_FACE ( 'NONE', ( #10852 ), #12949, .F. ) ;
#14210=FACE_OUTER_BOUND ( 'NONE', #11857, .T. ) ;
#14213=AXIS2_PLACEMENT_3D ( 'NONE', #13116, #14626, #823 ) ;
#14218=CIRCLE ( 'NONE', #9109, 9.000000000000001776 ) ;
#14231=FACE_OUTER_BOUND ( 'NONE', #5186, .T. ) ;
#14235=EDGE_CURVE ( 'NONE', #6609, #5566, #13043, .T. ) ;
#14238=EDGE_LOOP ( 'NONE', ( #18886, #18081 ) ) ;
#14241=ORIENTED_EDGE ( 'NONE', *, *, #18752, .F. ) ;
#14244=CARTESIAN_POINT ( 'NONE',  ( -9.580134541264520465, -14.56230589874905235, 32.00000000000000000 ) ) ;
#14248=AXIS2_PLACEMENT_3D ( 'NONE', #17363, #11462, #2348 ) ;
#14260=EDGE_LOOP ( 'NONE', ( #9753, #11806, #2212, #9101 ) ) ;
#14261=DIRECTION ( 'NONE',  ( 1.000000000000000000, 0.000000000000000000, 0.000000000000000000 ) ) ;
#14263=ORIENTED_EDGE ( 'NONE', *, *, #3917, .T. ) ;
#14268=VERTEX_POINT ( 'NONE', #19043 ) ;
#14269=CARTESIAN_POINT ( 'NONE',  ( -18.96448111170889206, 1.130229351527647808, 32.00000000000000000 ) ) ;
#14278=VERTEX_POINT ( 'NONE', #12749 ) ;
#14280=CARTESIAN_POINT ( 'NONE',  ( 11.32184790671639263, 13.12143529358541016, -35.00000000000000000 ) ) ;
#14286=DIRECTION ( 'NONE',  ( -0.000000000000000000, -0.000000000000000000, 1.000000000000000000 ) ) ;
#14290=CIRCLE ( 'NONE', #17478, 1.000000000000002665 ) ;
#14297=DIRECTION ( 'NONE',  ( -0.000000000000000000, -0.000000000000000000, 1.000000000000000000 ) ) ;
#14300=CARTESIAN_POINT ( 'NONE',  ( -1.255998204157475318, -17.85806462366060288, -32.00000000000000000 ) ) ;
#14306=DIRECTION ( 'NONE',  ( -0.000000000000000000, -0.000000000000000000, 1.000000000000000000 ) ) ;
#14307=ORIENTED_EDGE ( 'NONE', *, *, #2761, .T. ) ;
#14315=ORIENTED_EDGE ( 'NONE', *, *, #7221, .F. ) ;
#14319=AXIS2_PLACEMENT_3D ( 'NONE', #16324, #14436, #6907 ) ;
#14320=CARTESIAN_POINT ( 'NONE',  ( 5.510910596163084625E-16, 18.00000000000000355, -35.00000000000000000 ) ) ;
#14326=ORIENTED_EDGE ( 'NONE', *, *, #12099, .T. ) ;
#14327=CYLINDRICAL_SURFACE ( 'NONE', #2885, 1.000000000000000000 ) ;
#14332=LINE ( 'NONE', #6707, #11407 ) ;
#14333=DIRECTION ( 'NONE',  ( 0.000000000000000000, 0.000000000000000000, 1.000000000000000000 ) ) ;
#14337=CARTESIAN_POINT ( 'NONE',  ( 10.58013454126452046, -14.56230589874905412, 35.00000000000000000 ) ) ;
#14339=EDGE_LOOP ( 'NONE', ( #2286, #454 ) ) ;
#14343=DIRECTION ( 'NONE',  ( -0.000000000000000000, -0.000000000000000000, 1.000000000000000000 ) ) ;
#14344=EDGE_CURVE ( 'NONE', #12535, #3914, #9861, .T. ) ;
#14345=AXIS2_PLACEMENT_3D ( 'NONE', #511, #402, #6481 ) ;
#14351=CARTESIAN_POINT ( 'NONE',  ( -15.19790265903627180, 9.644882309621941374, -32.00000000000000000 ) ) ;
#14356=DIRECTION ( 'NONE',  ( 0.000000000000000000, 0.000000000000000000, -1.000000000000000000 ) ) ;
#14374=DIRECTION ( 'NONE',  ( 0.000000000000000000, 0.000000000000000000, 1.000000000000000000 ) ) ;
#14379=VERTEX_POINT ( 'NONE', #4129 ) ;
#14381=AXIS2_PLACEMENT_3D ( 'NONE', #13637, #19733, #10738 ) ;
#14386=DIRECTION ( 'NONE',  ( 1.000000000000000000, 0.000000000000000000, 0.000000000000000000 ) ) ;
#14392=DIRECTION ( 'NONE',  ( 0.000000000000000000, 0.000000000000000000, 1.000000000000000000 ) ) ;
#14393=CYLINDRICAL_SURFACE ( 'NONE', #13450, 22.00000000000000355 ) ;
#14397=DIRECTION ( 'NONE',  ( -0.000000000000000000, -0.000000000000000000, 1.000000000000000000 ) ) ;
#14398=DIRECTION ( 'NONE',  ( 1.000000000000000000, 0.000000000000000000, 0.000000000000000000 ) ) ;
#14404=DIRECTION ( 'NONE',  ( 1.000000000000000000, 0.000000000000000000, 0.000000000000000000 ) ) ;
#14406=UNCERTAINTY_MEASURE_WITH_UNIT (LENGTH_MEASURE( 1.000000000000000082E-05 ), #17225, 'distance_accuracy_value', 'NONE');
#14410=CARTESIAN_POINT ( 'NONE',  ( -16.28688694438836038, -7.664027248171298545, -32.00000000000000000 ) ) ;
#14418=CARTESIAN_POINT ( 'NONE',  ( -8.671566133830875600, 15.77352024078954429, -32.00000000000000000 ) ) ;
#14424=LINE ( 'NONE', #5311, #3389 ) ;
#14427=ORIENTED_EDGE ( 'NONE', *, *, #11774, .T. ) ;
#14433=FACE_OUTER_BOUND ( 'NONE', #5027, .T. ) ;
#14436=DIRECTION ( 'NONE',  ( 0.000000000000000000, 0.000000000000000000, 1.000000000000000000 ) ) ;
#14439=FACE_BOUND ( 'NONE', #12646, .T. ) ;
#14441=AXIS2_PLACEMENT_3D ( 'NONE', #2712, #10339, #17544 ) ;
#14442=EDGE_LOOP ( 'NONE', ( #18855, #6730, #18361, #16537 ) ) ;
#14444=AXIS2_PLACEMENT_3D ( 'NONE', #14540, #15836, #2412 ) ;
#14452=VERTEX_POINT ( 'NONE', #6669 ) ;
#14467=ORIENTED_EDGE ( 'NONE', *, *, #4667, .F. ) ;
#14468=EDGE_CURVE ( 'NONE', #5313, #8529, #8161, .T. ) ;
#14473=EDGE_LOOP ( 'NONE', ( #11905, #8873, #19100, #18670 ) ) ;
#14478=CARTESIAN_POINT ( 'NONE',  ( -10.58013454126452224, -14.56230589874905235, -32.00000000000000000 ) ) ;
#14489=ORIENTED_EDGE ( 'NONE', *, *, #12667, .T. ) ;
#14491=CIRCLE ( 'NONE', #425, 22.00000000000000355 ) ;
#14494=DIRECTION ( 'NONE',  ( 1.000000000000000000, 0.000000000000000000, 0.000000000000000000 ) ) ;
#14497=CIRCLE ( 'NONE', #2979, 22.00000000000000355 ) ;
#14498=DIRECTION ( 'NONE',  ( 1.000000000000000000, 0.000000000000000000, 0.000000000000000000 ) ) ;
#14503=CARTESIAN_POINT ( 'NONE',  ( -17.11901729331276911, 5.562305898749051458, 35.00000000000000000 ) ) ;
#14508=DIRECTION ( 'NONE',  ( 1.000000000000000000, 0.000000000000000000, 0.000000000000000000 ) ) ;
#14509=AXIS2_PLACEMENT_3D ( 'NONE', #6393, #18620, #15625 ) ;
#14510=FACE_OUTER_BOUND ( 'NONE', #15669, .T. ) ;
#14513=CARTESIAN_POINT ( 'NONE',  ( -16.28688694438836038, -7.664027248171298545, -32.00000000000000000 ) ) ;
#14518=EDGE_LOOP ( 'NONE', ( #12698, #4249 ) ) ;
#14527=VECTOR ( 'NONE', #1845, 1000.000000000000000 ) ;
#14530=DIRECTION ( 'NONE',  ( 1.000000000000000000, 0.000000000000000000, 0.000000000000000000 ) ) ;
#14540=CARTESIAN_POINT ( 'NONE',  ( -6.626241948324210540, -16.73597674598852336, 32.00000000000000000 ) ) ;
#14544=CARTESIAN_POINT ( 'NONE',  ( 16.28688694438835327, -7.664027248171309203, 35.00000000000000000 ) ) ;
#14548=DIRECTION ( 'NONE',  ( 1.000000000000000000, 0.000000000000000000, 0.000000000000000000 ) ) ;
#14550=EDGE_LOOP ( 'NONE', ( #5507, #3648 ) ) ;
#14551=CARTESIAN_POINT ( 'NONE',  ( 17.68117051311639898, -3.372863662543048591, -32.00000000000000000 ) ) ;
#14553=FACE_BOUND ( 'NONE', #12196, .T. ) ;
#14556=CARTESIAN_POINT ( 'NONE',  ( -2.255998204157477538, -17.85806462366060288, -35.00000000000000000 ) ) ;
#14560=DIRECTION ( 'NONE',  ( 0.000000000000000000, 0.000000000000000000, 1.000000000000000000 ) ) ;
#14562=CARTESIAN_POINT ( 'NONE',  ( 12.32184790671639618, 13.12143529358541016, 32.00000000000000000 ) ) ;
#14567=ORIENTED_EDGE ( 'NONE', *, *, #17366, .F. ) ;
#14578=EDGE_CURVE ( 'NONE', #6290, #12336, #9125, .T. ) ;
#14585=AXIS2_PLACEMENT_3D ( 'NONE', #14544, #5420, #10335 ) ;
#14590=DIRECTION ( 'NONE',  ( 0.000000000000000000, 0.000000000000000000, 1.000000000000000000 ) ) ;
#14602=CARTESIAN_POINT ( 'NONE',  ( 3.255998204157476206, -17.85806462366060288, 32.00000000000000000 ) ) ;
#14604=DIRECTION ( 'NONE',  ( 0.000000000000000000, 0.000000000000000000, 1.000000000000000000 ) ) ;
#14605=DIRECTION ( 'NONE',  ( -0.000000000000000000, -0.000000000000000000, 1.000000000000000000 ) ) ;
#14608=ADVANCED_FACE ( 'NONE', ( #13473 ), #15286, .F. ) ;
#14613=ORIENTED_EDGE ( 'NONE', *, *, #7683, .F. ) ;
#14616=EDGE_CURVE ( 'NONE', #8799, #15782, #14186, .T. ) ;
#14626=DIRECTION ( 'NONE',  ( 0.000000000000000000, 0.000000000000000000, 1.000000000000000000 ) ) ;
#14635=CYLINDRICAL_SURFACE ( 'NONE', #4834, 1.000000000000004441 ) ;
#14636=DIRECTION ( 'NONE',  ( -1.000000000000000000, 0.000000000000000000, 0.000000000000000000 ) ) ;
#14641=EDGE_LOOP ( 'NONE', ( #14467, #16976, #2487, #17945 ) ) ;
#14647=DIRECTION ( 'NONE',  ( 0.000000000000000000, 0.000000000000000000, -1.000000000000000000 ) ) ;
#14648=EDGE_CURVE ( 'NONE', #7726, #4563, #2399, .T. ) ;
#14650=PLANE ( 'NONE',  #13874 ) ;
#14652=DIRECTION ( 'NONE',  ( -0.000000000000000000, -0.000000000000000000, 1.000000000000000000 ) ) ;
#14657=DIRECTION ( 'NONE',  ( 0.000000000000000000, 0.000000000000000000, -1.000000000000000000 ) ) ;
#14661=CARTESIAN_POINT ( 'NONE',  ( 18.11901729331276911, 5.562305898749055011, -35.00000000000000000 ) ) ;
#14667=ORIENTED_EDGE ( 'NONE', *, *, #4243, .T. ) ;
#14673=DIRECTION ( 'NONE',  ( 1.000000000000000000, 0.000000000000000000, 0.000000000000000000 ) ) ;
#14677=EDGE_CURVE ( 'NONE', #3117, #3527, #6253, .T. ) ;
#14681=FACE_OUTER_BOUND ( 'NONE', #14641, .T. ) ;
#14685=EDGE_CURVE ( 'NONE', #5172, #9689, #4471, .T. ) ;
#14686=DIRECTION ( 'NONE',  ( 1.000000000000000000, 0.000000000000000000, 0.000000000000000000 ) ) ;
#14695=CARTESIAN_POINT ( 'NONE',  ( -5.476417968967388639, 17.43449690031536292, 32.00000000000000000 ) ) ;
#14715=ORIENTED_EDGE ( 'NONE', *, *, #18190, .T. ) ;
#14716=CARTESIAN_POINT ( 'NONE',  ( 11.32184790671639263, 13.12143529358541016, 32.00000000000000000 ) ) ;
#14720=VERTEX_POINT ( 'NONE', #4867 ) ;
#14722=VERTEX_POINT ( 'NONE', #9785 ) ;
#14731=DIRECTION ( 'NONE',  ( 0.000000000000000000, 0.000000000000000000, -1.000000000000000000 ) ) ;
#14738=ORIENTED_EDGE ( 'NONE', *, *, #4174, .F. ) ;
#14740=CARTESIAN_POINT ( 'NONE',  ( -13.86923836996420967, -11.47363181547641275, 32.00000000000000000 ) ) ;
#14741=FACE_BOUND ( 'NONE', #13027, .T. ) ;
#14743=FACE_OUTER_BOUND ( 'NONE', #3325, .T. ) ;
#14749=CARTESIAN_POINT ( 'NONE',  ( 2.255998204157473097, -17.85806462366060288, 35.00000000000000000 ) ) ;
#14753=AXIS2_PLACEMENT_3D ( 'NONE', #17856, #4151, #5837 ) ;
#14763=CARTESIAN_POINT ( 'NONE',  ( 2.255998204157473097, -17.85806462366060288, 32.00000000000000000 ) ) ;
#14764=ORIENTED_EDGE ( 'NONE', *, *, #1827, .F. ) ;
#14765=DIRECTION ( 'NONE',  ( 0.000000000000000000, 0.000000000000000000, 1.000000000000000000 ) ) ;
#14767=EDGE_CURVE ( 'NONE', #12820, #10790, #3011, .T. ) ;
#14770=ORIENTED_EDGE ( 'NONE', *, *, #7936, .F. ) ;
#14771=CARTESIAN_POINT ( 'NONE',  ( 8.671566133830875600, 15.77352024078954784, 32.00000000000000000 ) ) ;
#14776=CIRCLE ( 'NONE', #5807, 9.000000000000000000 ) ;
#14778=CARTESIAN_POINT ( 'NONE',  ( 1.000000000000003331, 18.00000000000000355, -32.00000000000000000 ) ) ;
#14783=VECTOR ( 'NONE', #5264, 1000.000000000000000 ) ;
#14784=ADVANCED_FACE ( 'NONE', ( #360, #12675, #16981, #15673, #574, #6645, #8164, #9576, #10975, #5061, #18869, #6444, #17270, #7955, #5153, #3264, #9380, #1769, #15576, #264, #1962, #3660, #3368, #6348, #8057, #17078, #9479 ), #1866, .F. ) ;
#14785=CYLINDRICAL_SURFACE ( 'NONE', #4875, 1.000000000000002665 ) ;
#14788=CIRCLE ( 'NONE', #15423, 0.9999999999999974465 ) ;
#14792=EDGE_CURVE ( 'NONE', #3914, #9386, #2676, .T. ) ;
#14803=EDGE_LOOP ( 'NONE', ( #1006, #5811 ) ) ;
#14807=DIRECTION ( 'NONE',  ( 1.000000000000000000, 0.000000000000000000, 0.000000000000000000 ) ) ;
#14808=ADVANCED_FACE ( 'NONE', ( #15972 ), #10169, .F. ) ;
#14812=EDGE_CURVE ( 'NONE', #2723, #10856, #10693, .T. ) ;
#14816=ORIENTED_EDGE ( 'NONE', *, *, #9573, .F. ) ;
#14828=CARTESIAN_POINT ( 'NONE',  ( 0.000000000000000000, 0.000000000000000000, -35.00000000000000000 ) ) ;
#14831=EDGE_CURVE ( 'NONE', #3527, #10068, #8762, .T. ) ;
#14839=ORIENTED_EDGE ( 'NONE', *, *, #10828, .F. ) ;
#14841=ORIENTED_EDGE ( 'NONE', *, *, #8569, .F. ) ;
#14849=CYLINDRICAL_SURFACE ( 'NONE', #6552, 1.000000000000000888 ) ;
#14854=CARTESIAN_POINT ( 'NONE',  ( -12.32184790671639085, 13.12143529358541549, -32.00000000000000000 ) ) ;
#14855=CIRCLE ( 'NONE', #13898, 1.000000000000002665 ) ;
#14858=CARTESIAN_POINT ( 'NONE',  ( 0.000000000000000000, 0.000000000000000000, -32.00000000000000000 ) ) ;
#14861=LINE ( 'NONE', #5354, #4127 ) ;
#14868=EDGE_LOOP ( 'NONE', ( #13171, #5457, #6723, #12672 ) ) ;
#14869=ORIENTED_EDGE ( 'NONE', *, *, #8974, .T. ) ;
#14870=CARTESIAN_POINT ( 'NONE',  ( -4.476417968967385974, 17.43449690031536292, -32.00000000000000000 ) ) ;
#14875=ORIENTED_EDGE ( 'NONE', *, *, #11015, .F. ) ;
#14887=AXIS2_PLACEMENT_3D ( 'NONE', #9540, #9339, #133 ) ;
#14897=DIRECTION ( 'NONE',  ( -1.000000000000000000, 0.000000000000000000, 0.000000000000000000 ) ) ;
#14903=DIRECTION ( 'NONE',  ( 1.000000000000000000, 0.000000000000000000, 0.000000000000000000 ) ) ;
#14905=VECTOR ( 'NONE', #5564, 1000.000000000000000 ) ;
#14917=FACE_OUTER_BOUND ( 'NONE', #8316, .T. ) ;
#14918=CIRCLE ( 'NONE', #5651, 14.00000000000000178 ) ;
#14921=EDGE_CURVE ( 'NONE', #17528, #226, #11959, .T. ) ;
#14923=CARTESIAN_POINT ( 'NONE',  ( 16.19790265903627358, 9.644882309621939598, -32.00000000000000000 ) ) ;
#14926=CARTESIAN_POINT ( 'NONE',  ( 17.96448111170888851, 1.130229351527639148, -32.00000000000000000 ) ) ;
#14932=ORIENTED_EDGE ( 'NONE', *, *, #7263, .T. ) ;
#14940=EDGE_LOOP ( 'NONE', ( #2578, #10793 ) ) ;
#14941=CARTESIAN_POINT ( 'NONE',  ( 11.58013454126452579, -14.56230589874905412, 35.00000000000000000 ) ) ;
#14947=VECTOR ( 'NONE', #8128, 1000.000000000000000 ) ;
#14948=EDGE_LOOP ( 'NONE', ( #5991, #129, #30, #6570 ) ) ;
#14949=DIRECTION ( 'NONE',  ( -0.000000000000000000, -0.000000000000000000, 1.000000000000000000 ) ) ;
#14950=LINE ( 'NONE', #19155, #17423 ) ;
#14951=ADVANCED_FACE ( 'NONE', ( #10662 ), #13355, .F. ) ;
#14957=DIRECTION ( 'NONE',  ( 1.000000000000000000, 0.000000000000000000, 0.000000000000000000 ) ) ;
#14959=EDGE_CURVE ( 'NONE', #17830, #4563, #7642, .T. ) ;
#14965=DIRECTION ( 'NONE',  ( 1.000000000000000000, 0.000000000000000000, 0.000000000000000000 ) ) ;
#14967=ORIENTED_EDGE ( 'NONE', *, *, #16066, .F. ) ;
#14968=DIRECTION ( 'NONE',  ( 1.000000000000000000, 0.000000000000000000, 0.000000000000000000 ) ) ;
#14970=CARTESIAN_POINT ( 'NONE',  ( -9.671566133830877376, 15.77352024078954429, -35.00000000000000000 ) ) ;
#14971=EDGE_CURVE ( 'NONE', #15645, #4507, #5042, .T. ) ;
#14972=ORIENTED_EDGE ( 'NONE', *, *, #11993, .T. ) ;
#14984=CIRCLE ( 'NONE', #933, 1.000000000000004441 ) ;
#14990=FACE_BOUND ( 'NONE', #14339, .T. ) ;
#14998=DIRECTION ( 'NONE',  ( 0.000000000000000000, 0.000000000000000000, 1.000000000000000000 ) ) ;
#15000=CIRCLE ( 'NONE', #3166, 1.000000000000002665 ) ;
#15005=CARTESIAN_POINT ( 'NONE',  ( 18.96448111170889206, 1.130229351527639148, 32.00000000000000000 ) ) ;
#15007=EDGE_CURVE ( 'NONE', #6004, #6940, #18849, .T. ) ;
#15008=ORIENTED_EDGE ( 'NONE', *, *, #18742, .F. ) ;
#15016=DIRECTION ( 'NONE',  ( 0.000000000000000000, 0.000000000000000000, -1.000000000000000000 ) ) ;
#15031=CIRCLE ( 'NONE', #16304, 1.000000000000000000 ) ;
#15035=EDGE_LOOP ( 'NONE', ( #10043, #1650 ) ) ;
#15039=VERTEX_POINT ( 'NONE', #17061 ) ;
#15042=DIRECTION ( 'NONE',  ( 0.000000000000000000, 0.000000000000000000, -1.000000000000000000 ) ) ;
#15043=CARTESIAN_POINT ( 'NONE',  ( -10.58013454126452224, -14.56230589874905235, -35.00000000000000000 ) ) ;
#15050=EDGE_LOOP ( 'NONE', ( #3922, #15758 ) ) ;
#15051=LINE ( 'NONE', #4445, #11856 ) ;
#15055=ORIENTED_EDGE ( 'NONE', *, *, #13411, .F. ) ;
#15056=DIRECTION ( 'NONE',  ( 0.000000000000000000, 0.000000000000000000, 1.000000000000000000 ) ) ;
#15065=AXIS2_PLACEMENT_3D ( 'NONE', #8458, #16164, #4141 ) ;
#15066=ORIENTED_EDGE ( 'NONE', *, *, #10242, .F. ) ;
#15072=DIRECTION ( 'NONE',  ( 1.000000000000000000, 0.000000000000000000, 0.000000000000000000 ) ) ;
#15073=ORIENTED_EDGE ( 'NONE', *, *, #13778, .F. ) ;
#15074=CARTESIAN_POINT ( 'NONE',  ( 5.476417968967387750, 17.43449690031536292, 35.00000000000000000 ) ) ;
#15077=AXIS2_PLACEMENT_3D ( 'NONE', #3013, #15332, #2907 ) ;
#15080=AXIS2_PLACEMENT_3D ( 'NONE', #108, #10913, #12118 ) ;
#15085=ORIENTED_EDGE ( 'NONE', *, *, #14792, .T. ) ;
#15086=CARTESIAN_POINT ( 'NONE',  ( -18.96448111170889206, 1.130229351527647585, -32.00000000000000000 ) ) ;
#15087=CYLINDRICAL_SURFACE ( 'NONE', #10306, 1.000000000000000888 ) ;
#15089=FACE_OUTER_BOUND ( 'NONE', #1445, .T. ) ;
#15090=AXIS2_PLACEMENT_3D ( 'NONE', #13601, #12106, #1983 ) ;
#15091=FACE_BOUND ( 'NONE', #7975, .T. ) ;
#15092=AXIS2_PLACEMENT_3D ( 'NONE', #15889, #14590, #6558 ) ;
#15095=CARTESIAN_POINT ( 'NONE',  ( 17.11901729331276556, 5.562305898749055011, -32.00000000000000000 ) ) ;
#15108=VERTEX_POINT ( 'NONE', #18549 ) ;
#15111=CYLINDRICAL_SURFACE ( 'NONE', #18990, 1.000000000000000888 ) ;
#15113=DIRECTION ( 'NONE',  ( 0.000000000000000000, 0.000000000000000000, -1.000000000000000000 ) ) ;
#15114=ORIENTED_EDGE ( 'NONE', *, *, #5596, .T. ) ;
#15119=CYLINDRICAL_SURFACE ( 'NONE', #1666, 0.9999999999999974465 ) ;
#15120=FACE_OUTER_BOUND ( 'NONE', #18772, .T. ) ;
#15132=DIRECTION ( 'NONE',  ( -1.000000000000000000, 0.000000000000000000, 0.000000000000000000 ) ) ;
#15135=CARTESIAN_POINT ( 'NONE',  ( 0.000000000000000000, 0.000000000000000000, -30.00000000000000355 ) ) ;
#15136=ORIENTED_EDGE ( 'NONE', *, *, #10006, .F. ) ;
#15138=VERTEX_POINT ( 'NONE', #11736 ) ;
#15148=CARTESIAN_POINT ( 'NONE',  ( -5.626241948324210540, -16.73597674598852336, 32.00000000000000000 ) ) ;
#15155=CARTESIAN_POINT ( 'NONE',  ( 0.000000000000000000, 0.000000000000000000, 35.00000000000000000 ) ) ;
#15160=VECTOR ( 'NONE', #16685, 1000.000000000000000 ) ;
#15165=ORIENTED_EDGE ( 'NONE', *, *, #17755, .T. ) ;
#15170=ADVANCED_FACE ( 'NONE', ( #14743 ), #5240, .F. ) ;
#15177=ORIENTED_EDGE ( 'NONE', *, *, #5206, .F. ) ;
#15178=EDGE_CURVE ( 'NONE', #155, #3939, #11960, .T. ) ;
#15182=ORIENTED_EDGE ( 'NONE', *, *, #9030, .T. ) ;
#15183=DIRECTION ( 'NONE',  ( 1.000000000000000000, 0.000000000000000000, 0.000000000000000000 ) ) ;
#15184=DIRECTION ( 'NONE',  ( -1.000000000000000000, 0.000000000000000000, 0.000000000000000000 ) ) ;
#15203=EDGE_CURVE ( 'NONE', #3148, #6388, #9752, .T. ) ;
#15204=EDGE_CURVE ( 'NONE', #5957, #4210, #5878, .T. ) ;
#15208=LINE ( 'NONE', #15005, #5494 ) ;
#15215=EDGE_LOOP ( 'NONE', ( #3411, #12780 ) ) ;
#15216=CARTESIAN_POINT ( 'NONE',  ( -12.86923836996420611, -11.47363181547641275, -32.00000000000000000 ) ) ;
#15223=AXIS2_PLACEMENT_3D ( 'NONE', #14740, #17835, #10143 ) ;
#15225=EDGE_CURVE ( 'NONE', #2419, #17102, #12294, .T. ) ;
#15227=ORIENTED_EDGE ( 'NONE', *, *, #3106, .T. ) ;
#15230=ORIENTED_EDGE ( 'NONE', *, *, #18090, .T. ) ;
#15234=ORIENTED_EDGE ( 'NONE', *, *, #11409, .T. ) ;
#15244=ORIENTED_EDGE ( 'NONE', *, *, #4982, .F. ) ;
#15245=CARTESIAN_POINT ( 'NONE',  ( 17.28688694438834972, -7.664027248171309203, 32.00000000000000000 ) ) ;
#15246=DIRECTION ( 'NONE',  ( 0.000000000000000000, 0.000000000000000000, 1.000000000000000000 ) ) ;
#15247=FACE_BOUND ( 'NONE', #4956, .T. ) ;
#15256=VECTOR ( 'NONE', #2025, 1000.000000000000000 ) ;
#15262=CARTESIAN_POINT ( 'NONE',  ( -17.68117051311639898, -3.372863662543042818, -32.00000000000000000 ) ) ;
#15266=CIRCLE ( 'NONE', #16551, 1.000000000000004441 ) ;
#15270=CARTESIAN_POINT ( 'NONE',  ( -2.255998204157477538, -17.85806462366060288, -32.00000000000000000 ) ) ;
#15271=EDGE_LOOP ( 'NONE', ( #12411, #4392, #6662, #11874 ) ) ;
#15286=CYLINDRICAL_SURFACE ( 'NONE', #9079, 12.00000000000000178 ) ;
#15287=EDGE_LOOP ( 'NONE', ( #2795, #2949 ) ) ;
#15290=CARTESIAN_POINT ( 'NONE',  ( 13.86923836996420789, -11.47363181547641453, -35.00000000000000000 ) ) ;
#15291=ORIENTED_EDGE ( 'NONE', *, *, #6616, .F. ) ;
#15294=FACE_BOUND ( 'NONE', #15616, .T. ) ;
#15296=EDGE_CURVE ( 'NONE', #4507, #8343, #4474, .T. ) ;
#15298=DIRECTION ( 'NONE',  ( 0.000000000000000000, 0.000000000000000000, 1.000000000000000000 ) ) ;
#15300=ORIENTED_EDGE ( 'NONE', *, *, #2266, .F. ) ;
#15308=LINE ( 'NONE', #8902, #18595 ) ;
#15310=ORIENTED_EDGE ( 'NONE', *, *, #2097, .F. ) ;
#15311=DIRECTION ( 'NONE',  ( 1.000000000000000000, 0.000000000000000000, 0.000000000000000000 ) ) ;
#15313=CARTESIAN_POINT ( 'NONE',  ( -16.28688694438836038, -7.664027248171298545, 32.00000000000000000 ) ) ;
#15314=EDGE_LOOP ( 'NONE', ( #14031, #188 ) ) ;
#15323=AXIS2_PLACEMENT_3D ( 'NONE', #18355, #17153, #12556 ) ;
#15329=ORIENTED_EDGE ( 'NONE', *, *, #11247, .F. ) ;
#15332=DIRECTION ( 'NONE',  ( -0.000000000000000000, -0.000000000000000000, 1.000000000000000000 ) ) ;
#15341=EDGE_LOOP ( 'NONE', ( #18056, #9532, #12152, #9302 ) ) ;
#15354=VERTEX_POINT ( 'NONE', #21 ) ;
#15358=FACE_OUTER_BOUND ( 'NONE', #6418, .T. ) ;
#15361=SURFACE_SIDE_STYLE ('',( #3043 ) ) ;
#15374=ORIENTED_EDGE ( 'NONE', *, *, #10549, .T. ) ;
#15376=ORIENTED_EDGE ( 'NONE', *, *, #12490, .T. ) ;
#15389=CYLINDRICAL_SURFACE ( 'NONE', #3102, 1.000000000000000888 ) ;
#15391=CYLINDRICAL_SURFACE ( 'NONE', #4546, 1.000000000000002442 ) ;
#15394=AXIS2_PLACEMENT_3D ( 'NONE', #16009, #11600, #17704 ) ;
#15395=ORIENTED_EDGE ( 'NONE', *, *, #7936, .T. ) ;
#15396=EDGE_CURVE ( 'NONE', #16380, #13666, #5734, .T. ) ;
#15405=CIRCLE ( 'NONE', #15090, 1.000000000000003109 ) ;
#15408=DIRECTION ( 'NONE',  ( 0.000000000000000000, 0.000000000000000000, 1.000000000000000000 ) ) ;
#15416=VERTEX_POINT ( 'NONE', #17942 ) ;
#15419=ORIENTED_EDGE ( 'NONE', *, *, #6250, .T. ) ;
#15423=AXIS2_PLACEMENT_3D ( 'NONE', #15897, #14397, #2180 ) ;
#15425=AXIS2_PLACEMENT_3D ( 'NONE', #13967, #258, #13572 ) ;
#15426=AXIS2_PLACEMENT_3D ( 'NONE', #18581, #19689, #6072 ) ;
#15431=ORIENTED_EDGE ( 'NONE', *, *, #8634, .T. ) ;
#15434=EDGE_LOOP ( 'NONE', ( #7831, #9518, #4460, #4014 ) ) ;
#15436=ORIENTED_EDGE ( 'NONE', *, *, #2557, .F. ) ;
#15442=ADVANCED_FACE ( 'NONE', ( #421 ), #18334, .F. ) ;
#15444=VECTOR ( 'NONE', #3532, 1000.000000000000000 ) ;
#15447=VECTOR ( 'NONE', #1509, 1000.000000000000000 ) ;
#15451=ADVANCED_FACE ( 'NONE', ( #9533 ), #4822, .F. ) ;
#15455=CARTESIAN_POINT ( 'NONE',  ( 17.28688694438834972, -7.664027248171309203, -35.00000000000000000 ) ) ;
#15467=ORIENTED_EDGE ( 'NONE', *, *, #14468, .T. ) ;
#15471=ORIENTED_EDGE ( 'NONE', *, *, #15203, .T. ) ;
#15475=ORIENTED_EDGE ( 'NONE', *, *, #8822, .T. ) ;
#15489=DIRECTION ( 'NONE',  ( 1.000000000000000000, 0.000000000000000000, 0.000000000000000000 ) ) ;
#15491=DIRECTION ( 'NONE',  ( 1.000000000000000000, 0.000000000000000000, 0.000000000000000000 ) ) ;
#15495=ORIENTED_EDGE ( 'NONE', *, *, #8983, .F. ) ;
#15498=VERTEX_POINT ( 'NONE', #9436 ) ;
#15500=CIRCLE ( 'NONE', #6849, 1.000000000000000888 ) ;
#15514=DIRECTION ( 'NONE',  ( 1.000000000000000000, 0.000000000000000000, 0.000000000000000000 ) ) ;
#15521=CARTESIAN_POINT ( 'NONE',  ( 16.11901729331276556, 5.562305898749055011, -35.00000000000000000 ) ) ;
#15526=CARTESIAN_POINT ( 'NONE',  ( -16.68117051311640253, -3.372863662543042818, 32.00000000000000000 ) ) ;
#15527=CARTESIAN_POINT ( 'NONE',  ( -16.28688694438836038, -7.664027248171298545, 35.00000000000000000 ) ) ;
#15534=ORIENTED_EDGE ( 'NONE', *, *, #13869, .F. ) ;
#15537=AXIS2_PLACEMENT_3D ( 'NONE', #5013, #6304, #17224 ) ;
#15542=CYLINDRICAL_SURFACE ( 'NONE', #11682, 1.000000000000002665 ) ;
#15559=DIRECTION ( 'NONE',  ( 1.000000000000000000, 0.000000000000000000, 0.000000000000000000 ) ) ;
#15562=VERTEX_POINT ( 'NONE', #11028 ) ;
#15572=AXIS2_PLACEMENT_3D ( 'NONE', #11812, #7491, #2997 ) ;
#15576=FACE_BOUND ( 'NONE', #656, .T. ) ;
#15580=DIRECTION ( 'NONE',  ( 0.000000000000000000, 0.000000000000000000, -1.000000000000000000 ) ) ;
#15582=EDGE_LOOP ( 'NONE', ( #6, #7579, #7598, #8635 ) ) ;
#15587=DIRECTION ( 'NONE',  ( 0.000000000000000000, 0.000000000000000000, 1.000000000000000000 ) ) ;
#15590=AXIS2_PLACEMENT_3D ( 'NONE', #8327, #833, #735 ) ;
#15595=DIRECTION ( 'NONE',  ( 1.000000000000000000, 0.000000000000000000, 0.000000000000000000 ) ) ;
#15597=CARTESIAN_POINT ( 'NONE',  ( -2.255998204157477538, -17.85806462366060288, 32.00000000000000000 ) ) ;
#15598=CARTESIAN_POINT ( 'NONE',  ( 17.68117051311639898, -3.372863662543048591, 32.00000000000000000 ) ) ;
#15603=CYLINDRICAL_SURFACE ( 'NONE', #5328, 1.000000000000000000 ) ;
#15605=AXIS2_PLACEMENT_3D ( 'NONE', #6292, #12418, #5004 ) ;
#15606=( NAMED_UNIT ( * ) SI_UNIT ( $, .STERADIAN. ) SOLID_ANGLE_UNIT ( ) );
#15607=EDGE_LOOP ( 'NONE', ( #17850, #18563, #8734, #2296 ) ) ;
#15613=VERTEX_POINT ( 'NONE', #10032 ) ;
#15614=CARTESIAN_POINT ( 'NONE',  ( -17.11901729331276911, 5.562305898749051458, 32.00000000000000000 ) ) ;
#15616=EDGE_LOOP ( 'NONE', ( #5909, #11986 ) ) ;
#15618=DIRECTION ( 'NONE',  ( 0.000000000000000000, 0.000000000000000000, 1.000000000000000000 ) ) ;
#15625=DIRECTION ( 'NONE',  ( -1.000000000000000000, 0.000000000000000000, 0.000000000000000000 ) ) ;
#15637=CARTESIAN_POINT ( 'NONE',  ( 8.671566133830875600, 15.77352024078954784, -32.00000000000000000 ) ) ;
#15640=ORIENTED_EDGE ( 'NONE', *, *, #13998, .T. ) ;
#15645=VERTEX_POINT ( 'NONE', #8221 ) ;
#15648=DIRECTION ( 'NONE',  ( 1.000000000000000000, 0.000000000000000000, 0.000000000000000000 ) ) ;
#15660=ORIENTED_EDGE ( 'NONE', *, *, #6826, .F. ) ;
#15669=EDGE_LOOP ( 'NONE', ( #4559, #15848, #19578, #11973 ) ) ;
#15673=FACE_BOUND ( 'NONE', #18509, .T. ) ;
#15686=DIRECTION ( 'NONE',  ( 1.000000000000000000, 0.000000000000000000, 0.000000000000000000 ) ) ;
#15694=CARTESIAN_POINT ( 'NONE',  ( -15.19790265903627180, 9.644882309621941374, -32.00000000000000000 ) ) ;
#15697=FACE_OUTER_BOUND ( 'NONE', #15434, .T. ) ;
#15699=CYLINDRICAL_SURFACE ( 'NONE', #12301, 0.9999999999999974465 ) ;
#15702=LINE ( 'NONE', #8092, #3772 ) ;
#15707=ADVANCED_FACE ( 'NONE', ( #8425 ), #14327, .F. ) ;
#15708=VECTOR ( 'NONE', #7518, 1000.000000000000000 ) ;
#15710=CARTESIAN_POINT ( 'NONE',  ( -7.671566133830872047, 15.77352024078954429, -32.00000000000000000 ) ) ;
#15713=CARTESIAN_POINT ( 'NONE',  ( 16.28688694438835327, -7.664027248171309203, -32.00000000000000000 ) ) ;
#15716=FACE_OUTER_BOUND ( 'NONE', #16576, .T. ) ;
#15720=VECTOR ( 'NONE', #733, 1000.000000000000000 ) ;
#15727=ORIENTED_EDGE ( 'NONE', *, *, #3337, .F. ) ;
#15731=ORIENTED_EDGE ( 'NONE', *, *, #8779, .T. ) ;
#15738=AXIS2_PLACEMENT_3D ( 'NONE', #2657, #13462, #4369 ) ;
#15741=AXIS2_PLACEMENT_3D ( 'NONE', #16698, #2980, #9094 ) ;
#15746=VECTOR ( 'NONE', #15580, 1000.000000000000000 ) ;
#15750=EDGE_LOOP ( 'NONE', ( #11616, #11843, #7647, #16543 ) ) ;
#15751=AXIS2_PLACEMENT_3D ( 'NONE', #17988, #10680, #16584 ) ;
#15758=ORIENTED_EDGE ( 'NONE', *, *, #8757, .T. ) ;
#15768=ORIENTED_EDGE ( 'NONE', *, *, #5115, .T. ) ;
#15773=CIRCLE ( 'NONE', #10352, 1.000000000000003553 ) ;
#15774=CYLINDRICAL_SURFACE ( 'NONE', #7094, 1.000000000000002665 ) ;
#15780=VERTEX_POINT ( 'NONE', #16515 ) ;
#15781=EDGE_CURVE ( 'NONE', #4160, #8143, #12476, .T. ) ;
#15782=VERTEX_POINT ( 'NONE', #11810 ) ;
#15789=ADVANCED_FACE ( 'NONE', ( #16416 ), #9009, .F. ) ;
#15800=CARTESIAN_POINT ( 'NONE',  ( 6.626241948324199882, -16.73597674598852691, 32.00000000000000000 ) ) ;
#15801=ORIENTED_EDGE ( 'NONE', *, *, #18017, .T. ) ;
#15813=CIRCLE ( 'NONE', #4624, 0.9999999999999974465 ) ;
#15819=CIRCLE ( 'NONE', #2690, 0.9999999999999974465 ) ;
#15825=CARTESIAN_POINT ( 'NONE',  ( 5.476417968967387750, 17.43449690031536292, -32.00000000000000000 ) ) ;
#15830=EDGE_CURVE ( 'NONE', #562, #13990, #7341, .T. ) ;
#15833=EDGE_CURVE ( 'NONE', #14379, #1977, #9410, .T. ) ;
#15836=DIRECTION ( 'NONE',  ( 0.000000000000000000, 0.000000000000000000, 1.000000000000000000 ) ) ;
#15839=CIRCLE ( 'NONE', #17759, 1.000000000000004441 ) ;
#15841=FACE_BOUND ( 'NONE', #16852, .T. ) ;
#15848=ORIENTED_EDGE ( 'NONE', *, *, #7878, .T. ) ;
#15850=DIRECTION ( 'NONE',  ( -1.000000000000000000, 0.000000000000000000, 0.000000000000000000 ) ) ;
#15852=DIRECTION ( 'NONE',  ( -0.000000000000000000, -0.000000000000000000, 1.000000000000000000 ) ) ;
#15864=CARTESIAN_POINT ( 'NONE',  ( 0.000000000000000000, 0.000000000000000000, -32.00000000000000000 ) ) ;
#15867=ORIENTED_EDGE ( 'NONE', *, *, #10864, .T. ) ;
#15871=ORIENTED_EDGE ( 'NONE', *, *, #13623, .T. ) ;
#15876=MANIFOLD_SOLID_BREP ( 'Boss-Extrude3', #7416 ) ;
#15880=LINE ( 'NONE', #6848, #14783 ) ;
#15882=CIRCLE ( 'NONE', #19697, 1.000000000000000888 ) ;
#15883=ORIENTED_EDGE ( 'NONE', *, *, #1710, .T. ) ;
#15884=ORIENTED_EDGE ( 'NONE', *, *, #11779, .T. ) ;
#15886=CARTESIAN_POINT ( 'NONE',  ( 12.00000000000000178, 1.469576158976824144E-15, 29.00000000000000355 ) ) ;
#15888=VERTEX_POINT ( 'NONE', #12608 ) ;
#15889=CARTESIAN_POINT ( 'NONE',  ( -4.476417968967385974, 17.43449690031536292, 35.00000000000000000 ) ) ;
#15891=AXIS2_PLACEMENT_3D ( 'NONE', #17944, #7514, #16447 ) ;
#15894=CIRCLE ( 'NONE', #5330, 1.000000000000004441 ) ;
#15897=CARTESIAN_POINT ( 'NONE',  ( -17.68117051311639898, -3.372863662543042818, -35.00000000000000000 ) ) ;
#15898=CYLINDRICAL_SURFACE ( 'NONE', #5558, 0.9999999999999974465 ) ;
#15904=ORIENTED_EDGE ( 'NONE', *, *, #9573, .T. ) ;
#15920=AXIS2_PLACEMENT_3D ( 'NONE', #15713, #3307, #6583 ) ;
#15926=ADVANCED_FACE ( 'NONE', ( #14510 ), #13358, .F. ) ;
#15927=ORIENTED_EDGE ( 'NONE', *, *, #17570, .T. ) ;
#15932=ORIENTED_EDGE ( 'NONE', *, *, #3560, .F. ) ;
#15937=AXIS2_PLACEMENT_3D ( 'NONE', #14870, #10569, #1163 ) ;
#15940=CARTESIAN_POINT ( 'NONE',  ( -16.28688694438836038, -7.664027248171298545, -32.00000000000000000 ) ) ;
#15944=FACE_OUTER_BOUND ( 'NONE', #16159, .T. ) ;
#15945=EDGE_CURVE ( 'NONE', #15354, #4315, #13122, .T. ) ;
#15947=FACE_OUTER_BOUND ( 'NONE', #12324, .T. ) ;
#15951=CARTESIAN_POINT ( 'NONE',  ( 22.00000000000000355, 2.694222958124177204E-15, -32.00000000000000000 ) ) ;
#15961=ORIENTED_EDGE ( 'NONE', *, *, #9879, .F. ) ;
#15963=DIRECTION ( 'NONE',  ( 0.000000000000000000, 0.000000000000000000, 1.000000000000000000 ) ) ;
#15965=VERTEX_POINT ( 'NONE', #11495 ) ;
#15966=AXIS2_PLACEMENT_3D ( 'NONE', #9782, #6346, #3366 ) ;
#15969=VERTEX_POINT ( 'NONE', #15996 ) ;
#15972=FACE_OUTER_BOUND ( 'NONE', #5119, .T. ) ;
#15973=ORIENTED_EDGE ( 'NONE', *, *, #8983, .T. ) ;
#15976=ORIENTED_EDGE ( 'NONE', *, *, #2785, .F. ) ;
#15982=DIRECTION ( 'NONE',  ( -0.000000000000000000, -0.000000000000000000, 1.000000000000000000 ) ) ;
#15989=CIRCLE ( 'NONE', #16952, 1.000000000000004441 ) ;
#15994=CYLINDRICAL_SURFACE ( 'NONE', #9167, 1.000000000000004441 ) ;
#15995=DIRECTION ( 'NONE',  ( 1.000000000000000000, 0.000000000000000000, 0.000000000000000000 ) ) ;
#15996=CARTESIAN_POINT ( 'NONE',  ( 3.255998204157476206, -17.85806462366060288, 35.00000000000000000 ) ) ;
#16006=AXIS2_PLACEMENT_3D ( 'NONE', #8310, #8415, #8699 ) ;
#16009=CARTESIAN_POINT ( 'NONE',  ( 16.28688694438835327, -7.664027248171309203, -32.00000000000000000 ) ) ;
#16011=VERTEX_POINT ( 'NONE', #5185 ) ;
#16018=AXIS2_PLACEMENT_3D ( 'NONE', #1545, #16955, #19651 ) ;
#16021=CARTESIAN_POINT ( 'NONE',  ( -8.671566133830875600, 15.77352024078954429, 35.00000000000000000 ) ) ;
#16025=ORIENTED_EDGE ( 'NONE', *, *, #6826, .T. ) ;
#16026=CARTESIAN_POINT ( 'NONE',  ( -16.68117051311640253, -3.372863662543042818, -32.00000000000000000 ) ) ;
#16035=CARTESIAN_POINT ( 'NONE',  ( 3.255998204157476206, -17.85806462366060288, -32.00000000000000000 ) ) ;
#16046=CARTESIAN_POINT ( 'NONE',  ( 16.96448111170888851, 1.130229351527639148, -32.00000000000000000 ) ) ;
#16049=FACE_BOUND ( 'NONE', #6146, .T. ) ;
#16053=CIRCLE ( 'NONE', #2302, 1.000000000000002665 ) ;
#16059=CARTESIAN_POINT ( 'NONE',  ( 16.96448111170888851, 1.130229351527639148, -32.00000000000000000 ) ) ;
#16060=ORIENTED_EDGE ( 'NONE', *, *, #7174, .F. ) ;
#16065=EDGE_LOOP ( 'NONE', ( #19638, #17719, #5337, #14241 ) ) ;
#16066=EDGE_CURVE ( 'NONE', #14722, #17321, #16278, .T. ) ;
#16072=VECTOR ( 'NONE', #5460, 1000.000000000000000 ) ;
#16075=EDGE_CURVE ( 'NONE', #12580, #6991, #10895, .T. ) ;
#16076=CIRCLE ( 'NONE', #17342, 1.000000000000004441 ) ;
#16092=VECTOR ( 'NONE', #1895, 1000.000000000000000 ) ;
#16094=ORIENTED_EDGE ( 'NONE', *, *, #15225, .T. ) ;
#16095=LINE ( 'NONE', #2177, #13273 ) ;
#16099=CARTESIAN_POINT ( 'NONE',  ( 18.96448111170889206, 1.130229351527639370, -32.00000000000000000 ) ) ;
#16100=CARTESIAN_POINT ( 'NONE',  ( -13.86923836996420967, -11.47363181547641275, -32.00000000000000000 ) ) ;
#16102=DIRECTION ( 'NONE',  ( 1.000000000000000000, 0.000000000000000000, 0.000000000000000000 ) ) ;
#16103=CARTESIAN_POINT ( 'NONE',  ( -4.476417968967385974, 17.43449690031536292, 32.00000000000000000 ) ) ;
#16104=CIRCLE ( 'NONE', #16746, 1.000000000000004441 ) ;
#16112=DIRECTION ( 'NONE',  ( 1.000000000000000000, 0.000000000000000000, 0.000000000000000000 ) ) ;
#16120=EDGE_LOOP ( 'NONE', ( #7439, #7984, #12461, #12500 ) ) ;
#16121=DIRECTION ( 'NONE',  ( 0.000000000000000000, 0.000000000000000000, -1.000000000000000000 ) ) ;
#16131=SHAPE_REPRESENTATION_RELATIONSHIP ( 'NONE' , 'NONE' ,  #13463, #12355 ) ;
#16134=ORIENTED_EDGE ( 'NONE', *, *, #14812, .F. ) ;
#16141=FACE_OUTER_BOUND ( 'NONE', #1260, .T. ) ;
#16151=ADVANCED_FACE ( 'NONE', ( #14052 ), #18554, .F. ) ;
#16155=FACE_BOUND ( 'NONE', #14550, .T. ) ;
#16158=CIRCLE ( 'NONE', #7826, 1.000000000000003109 ) ;
#16159=EDGE_LOOP ( 'NONE', ( #11002, #7712, #4786, #9411 ) ) ;
#16164=DIRECTION ( 'NONE',  ( -0.000000000000000000, -0.000000000000000000, 1.000000000000000000 ) ) ;
#16167=DIRECTION ( 'NONE',  ( 1.000000000000000000, 0.000000000000000000, 0.000000000000000000 ) ) ;
#16173=EDGE_LOOP ( 'NONE', ( #5454, #2173 ) ) ;
#16186=DIRECTION ( 'NONE',  ( 0.000000000000000000, 0.000000000000000000, -1.000000000000000000 ) ) ;
#16190=CARTESIAN_POINT ( 'NONE',  ( -2.255998204157477538, -17.85806462366060288, -35.00000000000000000 ) ) ;
#16195=ADVANCED_FACE ( 'NONE', ( #19148 ), #4140, .F. ) ;
#16203=DIRECTION ( 'NONE',  ( 1.000000000000000000, 0.000000000000000000, 0.000000000000000000 ) ) ;
#16214=DIRECTION ( 'NONE',  ( -1.000000000000000000, 0.000000000000000000, 0.000000000000000000 ) ) ;
#16218=ORIENTED_EDGE ( 'NONE', *, *, #18190, .F. ) ;
#16220=CARTESIAN_POINT ( 'NONE',  ( -16.68117051311640253, -3.372863662543042818, 32.00000000000000000 ) ) ;
#16227=DIRECTION ( 'NONE',  ( -1.000000000000000000, 0.000000000000000000, 0.000000000000000000 ) ) ;
#16230=ORIENTED_EDGE ( 'NONE', *, *, #74, .F. ) ;
#16235=CIRCLE ( 'NONE', #6629, 0.9999999999999974465 ) ;
#16237=DIRECTION ( 'NONE',  ( 1.000000000000000000, 0.000000000000000000, 0.000000000000000000 ) ) ;
#16238=FACE_OUTER_BOUND ( 'NONE', #16880, .T. ) ;
#16239=VERTEX_POINT ( 'NONE', #3748 ) ;
#16249=CARTESIAN_POINT ( 'NONE',  ( -1.000000000000001998, 18.00000000000000355, -32.00000000000000000 ) ) ;
#16252=DIRECTION ( 'NONE',  ( 1.000000000000000000, 0.000000000000000000, 0.000000000000000000 ) ) ;
#16268=ORIENTED_EDGE ( 'NONE', *, *, #286, .F. ) ;
#16271=VERTEX_POINT ( 'NONE', #5340 ) ;
#16273=CARTESIAN_POINT ( 'NONE',  ( -15.19790265903627180, 9.644882309621941374, 32.00000000000000000 ) ) ;
#16278=CIRCLE ( 'NONE', #14045, 1.000000000000002665 ) ;
#16286=EDGE_CURVE ( 'NONE', #7772, #3249, #3943, .T. ) ;
#16300=EDGE_CURVE ( 'NONE', #15416, #19054, #3186, .T. ) ;
#16304=AXIS2_PLACEMENT_3D ( 'NONE', #18579, #4778, #10885 ) ;
#16306=CYLINDRICAL_SURFACE ( 'NONE', #1765, 1.000000000000000888 ) ;
#16310=DIRECTION ( 'NONE',  ( 1.000000000000000000, 0.000000000000000000, 0.000000000000000000 ) ) ;
#16320=AXIS2_PLACEMENT_3D ( 'NONE', #15597, #17290, #3487 ) ;
#16321=( GEOMETRIC_REPRESENTATION_CONTEXT ( 3 ) GLOBAL_UNCERTAINTY_ASSIGNED_CONTEXT ( ( #2387 ) ) GLOBAL_UNIT_ASSIGNED_CONTEXT ( ( #7591, #17107, #15606 ) ) REPRESENTATION_CONTEXT ( 'NONE', 'WORKASPACE' ) );
#16324=CARTESIAN_POINT ( 'NONE',  ( -16.28688694438836038, -7.664027248171298545, 35.00000000000000000 ) ) ;
#16327=DIRECTION ( 'NONE',  ( -1.000000000000000000, 0.000000000000000000, 0.000000000000000000 ) ) ;
#16331=LINE ( 'NONE', #4125, #17950 ) ;
#16340=ORIENTED_EDGE ( 'NONE', *, *, #13998, .F. ) ;
#16344=LINE ( 'NONE', #2345, #19209 ) ;
#16349=CARTESIAN_POINT ( 'NONE',  ( 1.000000000000003331, 18.00000000000000355, 35.00000000000000000 ) ) ;
#16353=DIRECTION ( 'NONE',  ( 1.000000000000000000, 0.000000000000000000, 0.000000000000000000 ) ) ;
#16356=CARTESIAN_POINT ( 'NONE',  ( 10.58013454126452046, -14.56230589874905412, 32.00000000000000000 ) ) ;
#16357=AXIS2_PLACEMENT_3D ( 'NONE', #14320, #3709, #4915 ) ;
#16377=CARTESIAN_POINT ( 'NONE',  ( -11.32184790671638730, 13.12143529358541549, 32.00000000000000000 ) ) ;
#16378=VECTOR ( 'NONE', #1778, 1000.000000000000000 ) ;
#16380=VERTEX_POINT ( 'NONE', #14941 ) ;
#16381=DIRECTION ( 'NONE',  ( 0.000000000000000000, 0.000000000000000000, -1.000000000000000000 ) ) ;
#16392=DIRECTION ( 'NONE',  ( 1.000000000000000000, 0.000000000000000000, 0.000000000000000000 ) ) ;
#16411=CARTESIAN_POINT ( 'NONE',  ( 13.32184790671640151, 13.12143529358541016, -32.00000000000000000 ) ) ;
#16416=FACE_OUTER_BOUND ( 'NONE', #4798, .T. ) ;
#16424=ADVANCED_FACE ( 'NONE', ( #14231 ), #9639, .F. ) ;
#16431=FACE_OUTER_BOUND ( 'NONE', #8253, .T. ) ;
#16432=ORIENTED_EDGE ( 'NONE', *, *, #4521, .F. ) ;
#16434=AXIS2_PLACEMENT_3D ( 'NONE', #6945, #19162, #2359 ) ;
#16435=CARTESIAN_POINT ( 'NONE',  ( 12.32184790671639618, 13.12143529358541016, 35.00000000000000000 ) ) ;
#16441=ADVANCED_FACE ( 'NONE', ( #7720 ), #325, .F. ) ;
#16447=DIRECTION ( 'NONE',  ( 1.000000000000000000, 0.000000000000000000, 0.000000000000000000 ) ) ;
#16448=EDGE_LOOP ( 'NONE', ( #15467, #18629 ) ) ;
#16454=DIRECTION ( 'NONE',  ( 0.000000000000000000, 0.000000000000000000, 1.000000000000000000 ) ) ;
#16462=EDGE_CURVE ( 'NONE', #18644, #3152, #963, .T. ) ;
#16465=FACE_OUTER_BOUND ( 'NONE', #8506, .T. ) ;
#16467=EDGE_LOOP ( 'NONE', ( #11224, #8637 ) ) ;
#16479=CARTESIAN_POINT ( 'NONE',  ( -10.58013454126452224, -14.56230589874905235, -32.00000000000000000 ) ) ;
#16480=EDGE_LOOP ( 'NONE', ( #11174, #1167 ) ) ;
#16487=EDGE_CURVE ( 'NONE', #5305, #4629, #19477, .T. ) ;
#16491=LINE ( 'NONE', #10490, #6285 ) ;
#16494=AXIS2_PLACEMENT_3D ( 'NONE', #18324, #15618, #9824 ) ;
#16497=FACE_OUTER_BOUND ( 'NONE', #7050, .T. ) ;
#16500=ORIENTED_EDGE ( 'NONE', *, *, #13187, .F. ) ;
#16505=ORIENTED_EDGE ( 'NONE', *, *, #6861, .F. ) ;
#16515=CARTESIAN_POINT ( 'NONE',  ( 12.86923836996420967, -11.47363181547641453, 35.00000000000000000 ) ) ;
#16519=CIRCLE ( 'NONE', #2131, 1.000000000000000888 ) ;
#16526=CARTESIAN_POINT ( 'NONE',  ( 13.32184790671640151, 13.12143529358541016, -32.00000000000000000 ) ) ;
#16529=EDGE_CURVE ( 'NONE', #9896, #5740, #7321, .T. ) ;
#16531=ORIENTED_EDGE ( 'NONE', *, *, #13377, .T. ) ;
#16537=ORIENTED_EDGE ( 'NONE', *, *, #17312, .T. ) ;
#16539=CARTESIAN_POINT ( 'NONE',  ( 7.671566133830872047, 15.77352024078954784, -35.00000000000000000 ) ) ;
#16541=ORIENTED_EDGE ( 'NONE', *, *, #14616, .F. ) ;
#16542=DIRECTION ( 'NONE',  ( 0.000000000000000000, 0.000000000000000000, 1.000000000000000000 ) ) ;
#16543=ORIENTED_EDGE ( 'NONE', *, *, #16757, .F. ) ;
#16547=CARTESIAN_POINT ( 'NONE',  ( 0.000000000000000000, 0.000000000000000000, -35.00000000000000000 ) ) ;
#16550=FACE_OUTER_BOUND ( 'NONE', #6445, .T. ) ;
#16551=AXIS2_PLACEMENT_3D ( 'NONE', #8613, #17433, #8224 ) ;
#16554=ORIENTED_EDGE ( 'NONE', *, *, #6938, .T. ) ;
#16556=ADVANCED_FACE ( 'NONE', ( #14433 ), #8431, .F. ) ;
#16558=ORIENTED_EDGE ( 'NONE', *, *, #9301, .T. ) ;
#16561=VECTOR ( 'NONE', #9090, 1000.000000000000000 ) ;
#16566=DIRECTION ( 'NONE',  ( 1.000000000000000000, 0.000000000000000000, 0.000000000000000000 ) ) ;
#16567=EDGE_LOOP ( 'NONE', ( #11591, #10876 ) ) ;
#16569=VERTEX_POINT ( 'NONE', #4015 ) ;
#16573=ORIENTED_EDGE ( 'NONE', *, *, #17824, .F. ) ;
#16574=DIRECTION ( 'NONE',  ( 0.000000000000000000, 0.000000000000000000, 1.000000000000000000 ) ) ;
#16576=EDGE_LOOP ( 'NONE', ( #11579, #321, #6501, #11958 ) ) ;
#16577=CIRCLE ( 'NONE', #10820, 1.000000000000004441 ) ;
#16584=DIRECTION ( 'NONE',  ( 1.000000000000000000, 0.000000000000000000, 0.000000000000000000 ) ) ;
#16587=AXIS2_PLACEMENT_3D ( 'NONE', #15864, #8043, #5441 ) ;
#16592=CARTESIAN_POINT ( 'NONE',  ( 16.28688694438835327, -7.664027248171309203, 32.00000000000000000 ) ) ;
#16593=FACE_BOUND ( 'NONE', #15035, .T. ) ;
#16598=EDGE_CURVE ( 'NONE', #7172, #13172, #12151, .T. ) ;
#16600=LINE ( 'NONE', #13593, #10606 ) ;
#16608=ORIENTED_EDGE ( 'NONE', *, *, #3331, .F. ) ;
#16610=DIRECTION ( 'NONE',  ( 0.000000000000000000, 0.000000000000000000, -1.000000000000000000 ) ) ;
#16613=DIRECTION ( 'NONE',  ( 0.000000000000000000, 0.000000000000000000, 1.000000000000000000 ) ) ;
#16616=CARTESIAN_POINT ( 'NONE',  ( 16.28688694438835327, -7.664027248171309203, -32.00000000000000000 ) ) ;
#16617=AXIS2_PLACEMENT_3D ( 'NONE', #19215, #5508, #10037 ) ;
#16618=DIRECTION ( 'NONE',  ( -0.000000000000000000, -0.000000000000000000, 1.000000000000000000 ) ) ;
#16621=ORIENTED_EDGE ( 'NONE', *, *, #2467, .T. ) ;
#16640=EDGE_LOOP ( 'NONE', ( #17585, #15801 ) ) ;
#16647=DIRECTION ( 'NONE',  ( -1.000000000000000000, 0.000000000000000000, 0.000000000000000000 ) ) ;
#16649=VECTOR ( 'NONE', #6462, 1000.000000000000000 ) ;
#16673=VERTEX_POINT ( 'NONE', #17531 ) ;
#16677=DIRECTION ( 'NONE',  ( 0.000000000000000000, 0.000000000000000000, 1.000000000000000000 ) ) ;
#16680=AXIS2_PLACEMENT_3D ( 'NONE', #17899, #14998, #1290 ) ;
#16685=DIRECTION ( 'NONE',  ( 0.000000000000000000, 0.000000000000000000, -1.000000000000000000 ) ) ;
#16691=ORIENTED_EDGE ( 'NONE', *, *, #2097, .T. ) ;
#16694=FACE_BOUND ( 'NONE', #19161, .T. ) ;
#16695=AXIS2_PLACEMENT_3D ( 'NONE', #4859, #7552, #1470 ) ;
#16696=DIRECTION ( 'NONE',  ( 0.000000000000000000, 0.000000000000000000, -1.000000000000000000 ) ) ;
#16698=CARTESIAN_POINT ( 'NONE',  ( 6.626241948324199882, -16.73597674598852691, 35.00000000000000000 ) ) ;
#16700=VERTEX_POINT ( 'NONE', #5795 ) ;
#16703=EDGE_LOOP ( 'NONE', ( #15374, #15395 ) ) ;
#16705=ADVANCED_FACE ( 'NONE', ( #5698 ), #2698, .F. ) ;
#16712=ADVANCED_FACE ( 'NONE', ( #14917 ), #9115, .F. ) ;
#16716=EDGE_CURVE ( 'NONE', #5566, #4750, #9595, .T. ) ;
#16723=FACE_OUTER_BOUND ( 'NONE', #17163, .T. ) ;
#16724=AXIS2_PLACEMENT_3D ( 'NONE', #17428, #9833, #6230 ) ;
#16726=CARTESIAN_POINT ( 'NONE',  ( -11.58013454126452579, -14.56230589874905235, 32.00000000000000000 ) ) ;
#16731=AXIS2_PLACEMENT_3D ( 'NONE', #4091, #10103, #16203 ) ;
#16740=VERTEX_POINT ( 'NONE', #13510 ) ;
#16742=ORIENTED_EDGE ( 'NONE', *, *, #14685, .F. ) ;
#16746=AXIS2_PLACEMENT_3D ( 'NONE', #15527, #7907, #8516 ) ;
#16757=EDGE_CURVE ( 'NONE', #17855, #257, #13712, .T. ) ;
#16764=CYLINDRICAL_SURFACE ( 'NONE', #4567, 1.000000000000003109 ) ;
#16765=ORIENTED_EDGE ( 'NONE', *, *, #2662, .F. ) ;
#16767=LINE ( 'NONE', #1249, #5920 ) ;
#16770=ORIENTED_EDGE ( 'NONE', *, *, #8558, .T. ) ;
#16776=ORIENTED_EDGE ( 'NONE', *, *, #15830, .T. ) ;
#16785=ORIENTED_EDGE ( 'NONE', *, *, #11138, .F. ) ;
#16794=CARTESIAN_POINT ( 'NONE',  ( 6.626241948324199882, -16.73597674598852691, -32.00000000000000000 ) ) ;
#16805=ORIENTED_EDGE ( 'NONE', *, *, #17542, .T. ) ;
#16807=LINE ( 'NONE', #10792, #5952 ) ;
#16814=AXIS2_PLACEMENT_3D ( 'NONE', #3056, #6714, #1832 ) ;
#16820=DIRECTION ( 'NONE',  ( 0.000000000000000000, 0.000000000000000000, 1.000000000000000000 ) ) ;
#16830=VECTOR ( 'NONE', #14731, 1000.000000000000000 ) ;
#16834=ORIENTED_EDGE ( 'NONE', *, *, #7911, .T. ) ;
#16841=AXIS2_PLACEMENT_3D ( 'NONE', #4886, #9699, #17190 ) ;
#16844=ORIENTED_EDGE ( 'NONE', *, *, #11379, .F. ) ;
#16845=CARTESIAN_POINT ( 'NONE',  ( -3.476417968967383754, 17.43449690031536292, -32.00000000000000000 ) ) ;
#16852=EDGE_LOOP ( 'NONE', ( #11326, #15475 ) ) ;
#16853=CARTESIAN_POINT ( 'NONE',  ( -18.11901729331277267, 5.562305898749051458, 32.00000000000000000 ) ) ;
#16854=VECTOR ( 'NONE', #18243, 1000.000000000000000 ) ;
#16856=AXIS2_PLACEMENT_3D ( 'NONE', #15637, #9746, #4930 ) ;
#16865=AXIS2_PLACEMENT_3D ( 'NONE', #19120, #5599, #3719 ) ;
#16872=EDGE_CURVE ( 'NONE', #1230, #6609, #11522, .T. ) ;
#16878=DIRECTION ( 'NONE',  ( -1.000000000000000000, 0.000000000000000000, 0.000000000000000000 ) ) ;
#16880=EDGE_LOOP ( 'NONE', ( #19090, #15234, #6812, #17745 ) ) ;
#16882=DIRECTION ( 'NONE',  ( -1.000000000000000000, 0.000000000000000000, 0.000000000000000000 ) ) ;
#16884=DIRECTION ( 'NONE',  ( -0.000000000000000000, -0.000000000000000000, -1.000000000000000000 ) ) ;
#16892=ORIENTED_EDGE ( 'NONE', *, *, #1920, .T. ) ;
#16894=DIRECTION ( 'NONE',  ( 1.000000000000000000, 0.000000000000000000, -0.000000000000000000 ) ) ;
#16922=ORIENTED_EDGE ( 'NONE', *, *, #2107, .F. ) ;
#16924=CIRCLE ( 'NONE', #15966, 1.000000000000004441 ) ;
#16925=LINE ( 'NONE', #8204, #13676 ) ;
#16942=ORIENTED_EDGE ( 'NONE', *, *, #6650, .F. ) ;
#16943=AXIS2_PLACEMENT_3D ( 'NONE', #13837, #2024, #9440 ) ;
#16952=AXIS2_PLACEMENT_3D ( 'NONE', #11889, #1286, #18197 ) ;
#16953=VERTEX_POINT ( 'NONE', #5876 ) ;
#16954=AXIS2_PLACEMENT_3D ( 'NONE', #797, #8765, #5744 ) ;
#16955=DIRECTION ( 'NONE',  ( -0.000000000000000000, -0.000000000000000000, 1.000000000000000000 ) ) ;
#16965=EDGE_CURVE ( 'NONE', #3823, #2901, #19484, .T. ) ;
#16968=VERTEX_POINT ( 'NONE', #1484 ) ;
#16969=DIRECTION ( 'NONE',  ( 1.000000000000000000, 0.000000000000000000, 0.000000000000000000 ) ) ;
#16976=ORIENTED_EDGE ( 'NONE', *, *, #7596, .T. ) ;
#16979=DIRECTION ( 'NONE',  ( 0.000000000000000000, 0.000000000000000000, -1.000000000000000000 ) ) ;
#16981=FACE_BOUND ( 'NONE', #10361, .T. ) ;
#16984=CARTESIAN_POINT ( 'NONE',  ( -8.671566133830875600, 15.77352024078954429, 35.00000000000000000 ) ) ;
#16987=ORIENTED_EDGE ( 'NONE', *, *, #11494, .F. ) ;
#17001=EDGE_CURVE ( 'NONE', #9729, #15416, #17796, .T. ) ;
#17004=CARTESIAN_POINT ( 'NONE',  ( 17.11901729331276556, 5.562305898749055011, 35.00000000000000000 ) ) ;
#17005=DIRECTION ( 'NONE',  ( 0.000000000000000000, 0.000000000000000000, 1.000000000000000000 ) ) ;
#17006=EDGE_LOOP ( 'NONE', ( #459, #11199, #13665, #1124 ) ) ;
#17008=CIRCLE ( 'NONE', #16695, 1.000000000000000888 ) ;
#17009=CARTESIAN_POINT ( 'NONE',  ( -17.96448111170888851, 1.130229351527647585, 32.00000000000000000 ) ) ;
#17012=EDGE_LOOP ( 'NONE', ( #2671, #417 ) ) ;
#17026=CIRCLE ( 'NONE', #8055, 1.000000000000002665 ) ;
#17031=CARTESIAN_POINT ( 'NONE',  ( 0.000000000000000000, 0.000000000000000000, 35.00000000000000000 ) ) ;
#17036=EDGE_CURVE ( 'NONE', #3939, #155, #15989, .T. ) ;
#17037=DIRECTION ( 'NONE',  ( 1.000000000000000000, 0.000000000000000000, 0.000000000000000000 ) ) ;
#17050=CARTESIAN_POINT ( 'NONE',  ( 16.11901729331276556, 5.562305898749055011, 32.00000000000000000 ) ) ;
#17052=ORIENTED_EDGE ( 'NONE', *, *, #13095, .T. ) ;
#17054=DIRECTION ( 'NONE',  ( 1.000000000000000000, 0.000000000000000000, 0.000000000000000000 ) ) ;
#17057=CARTESIAN_POINT ( 'NONE',  ( -15.19790265903627180, 9.644882309621941374, 32.00000000000000000 ) ) ;
#17061=CARTESIAN_POINT ( 'NONE',  ( -7.626241948324210540, -16.73597674598852336, 32.00000000000000000 ) ) ;
#17071=EDGE_CURVE ( 'NONE', #5740, #9896, #2550, .T. ) ;
#17073=VECTOR ( 'NONE', #10827, 1000.000000000000000 ) ;
#17077=FACE_OUTER_BOUND ( 'NONE', #17457, .T. ) ;
#17078=FACE_BOUND ( 'NONE', #2846, .T. ) ;
#17080=CARTESIAN_POINT ( 'NONE',  ( 10.58013454126452046, -14.56230589874905412, 32.00000000000000000 ) ) ;
#17087=CARTESIAN_POINT ( 'NONE',  ( -14.86923836996421144, -11.47363181547641275, 32.00000000000000000 ) ) ;
#17088=EDGE_CURVE ( 'NONE', #15498, #7633, #15031, .T. ) ;
#17090=AXIS2_PLACEMENT_3D ( 'NONE', #14418, #11415, #16214 ) ;
#17095=ORIENTED_EDGE ( 'NONE', *, *, #9879, .T. ) ;
#17098=DIRECTION ( 'NONE',  ( -0.000000000000000000, -0.000000000000000000, 1.000000000000000000 ) ) ;
#17102=VERTEX_POINT ( 'NONE', #9287 ) ;
#17107=( NAMED_UNIT ( * ) PLANE_ANGLE_UNIT ( ) SI_UNIT ( $, .RADIAN. ) );
#17108=ORIENTED_EDGE ( 'NONE', *, *, #8182, .F. ) ;
#17117=CARTESIAN_POINT ( 'NONE',  ( 18.96448111170889206, 1.130229351527639370, -35.00000000000000000 ) ) ;
#17122=ORIENTED_EDGE ( 'NONE', *, *, #8478, .F. ) ;
#17147=VECTOR ( 'NONE', #11683, 1000.000000000000000 ) ;
#17148=CARTESIAN_POINT ( 'NONE',  ( 17.11901729331276556, 5.562305898749055011, -32.00000000000000000 ) ) ;
#17152=VERTEX_POINT ( 'NONE', #17087 ) ;
#17153=DIRECTION ( 'NONE',  ( 0.000000000000000000, 0.000000000000000000, 1.000000000000000000 ) ) ;
#17163=EDGE_LOOP ( 'NONE', ( #8671, #16805, #4202, #1182 ) ) ;
#17184=DIRECTION ( 'NONE',  ( 1.000000000000000000, 0.000000000000000000, 0.000000000000000000 ) ) ;
#17190=DIRECTION ( 'NONE',  ( -1.000000000000000000, 0.000000000000000000, 0.000000000000000000 ) ) ;
#17191=EDGE_LOOP ( 'NONE', ( #16541, #16608 ) ) ;
#17195=CYLINDRICAL_SURFACE ( 'NONE', #11572, 22.00000000000000355 ) ;
#17202=FACE_OUTER_BOUND ( 'NONE', #11521, .T. ) ;
#17214=ORIENTED_EDGE ( 'NONE', *, *, #3432, .T. ) ;
#17216=CARTESIAN_POINT ( 'NONE',  ( 4.476417968967386862, 17.43449690031536292, -32.00000000000000000 ) ) ;
#17217=AXIS2_PLACEMENT_3D ( 'NONE', #17750, #10154, #16252 ) ;
#17218=ORIENTED_EDGE ( 'NONE', *, *, #3331, .T. ) ;
#17223=ORIENTED_EDGE ( 'NONE', *, *, #19221, .T. ) ;
#17224=DIRECTION ( 'NONE',  ( -1.000000000000000000, 0.000000000000000000, 0.000000000000000000 ) ) ;
#17225=( LENGTH_UNIT ( ) NAMED_UNIT ( * ) SI_UNIT ( .MILLI., .METRE. ) );
#17237=ORIENTED_EDGE ( 'NONE', *, *, #17570, .F. ) ;
#17239=FACE_OUTER_BOUND ( 'NONE', #1728, .T. ) ;
#17241=CARTESIAN_POINT ( 'NONE',  ( -7.671566133830872047, 15.77352024078954429, 32.00000000000000000 ) ) ;
#17251=EDGE_CURVE ( 'NONE', #18074, #16953, #5839, .T. ) ;
#17270=FACE_BOUND ( 'NONE', #19462, .T. ) ;
#17281=DIRECTION ( 'NONE',  ( 0.000000000000000000, 0.000000000000000000, 1.000000000000000000 ) ) ;
#17289=CARTESIAN_POINT ( 'NONE',  ( 17.11901729331276556, 5.562305898749055011, 35.00000000000000000 ) ) ;
#17290=DIRECTION ( 'NONE',  ( 0.000000000000000000, 0.000000000000000000, 1.000000000000000000 ) ) ;
#17291=EDGE_CURVE ( 'NONE', #4727, #14720, #10364, .T. ) ;
#17294=FACE_OUTER_BOUND ( 'NONE', #177, .T. ) ;
#17301=AXIS2_PLACEMENT_3D ( 'NONE', #18254, #143, #2932 ) ;
#17306=DIRECTION ( 'NONE',  ( 1.000000000000000000, 0.000000000000000000, 0.000000000000000000 ) ) ;
#17312=EDGE_CURVE ( 'NONE', #19582, #6940, #8007, .T. ) ;
#17315=ADVANCED_FACE ( 'NONE', ( #19654 ), #18163, .F. ) ;
#17317=CIRCLE ( 'NONE', #2925, 1.000000000000000888 ) ;
#17321=VERTEX_POINT ( 'NONE', #19108 ) ;
#17322=LINE ( 'NONE', #3712, #8831 ) ;
#17324=DIRECTION ( 'NONE',  ( 1.000000000000000000, 0.000000000000000000, 0.000000000000000000 ) ) ;
#17325=AXIS2_PLACEMENT_3D ( 'NONE', #15290, #2668, #7665 ) ;
#17329=CARTESIAN_POINT ( 'NONE',  ( -12.32184790671639085, 13.12143529358541549, 35.00000000000000000 ) ) ;
#17338=AXIS2_PLACEMENT_3D ( 'NONE', #7670, #15298, #4879 ) ;
#17339=FACE_BOUND ( 'NONE', #13233, .T. ) ;
#17342=AXIS2_PLACEMENT_3D ( 'NONE', #12163, #10272, #10565 ) ;
#17343=DIRECTION ( 'NONE',  ( -0.000000000000000000, -0.000000000000000000, 1.000000000000000000 ) ) ;
#17348=ORIENTED_EDGE ( 'NONE', *, *, #7969, .F. ) ;
#17363=CARTESIAN_POINT ( 'NONE',  ( -6.626241948324210540, -16.73597674598852336, 32.00000000000000000 ) ) ;
#17366=EDGE_CURVE ( 'NONE', #5957, #18333, #19200, .T. ) ;
#17368=PRODUCT ( 'Outer Wheel Hub Shell', 'Outer Wheel Hub Shell', '', ( #1651 ) ) ;
#17371=EDGE_CURVE ( 'NONE', #9559, #15354, #10212, .T. ) ;
#17376=EDGE_LOOP ( 'NONE', ( #2165, #14932 ) ) ;
#17381=CARTESIAN_POINT ( 'NONE',  ( 18.68117051311639543, -3.372863662543048591, -35.00000000000000000 ) ) ;
#17387=DIRECTION ( 'NONE',  ( -0.000000000000000000, -0.000000000000000000, 1.000000000000000000 ) ) ;
#17394=EDGE_CURVE ( 'NONE', #7691, #15645, #6395, .T. ) ;
#17396=CIRCLE ( 'NONE', #6519, 0.9999999999999974465 ) ;
#17397=DIRECTION ( 'NONE',  ( 1.000000000000000000, 0.000000000000000000, 0.000000000000000000 ) ) ;
#17401=DIRECTION ( 'NONE',  ( 1.000000000000000000, 0.000000000000000000, 0.000000000000000000 ) ) ;
#17410=DIRECTION ( 'NONE',  ( 0.000000000000000000, 0.000000000000000000, 1.000000000000000000 ) ) ;
#17419=CYLINDRICAL_SURFACE ( 'NONE', #8835, 1.000000000000004441 ) ;
#17420=ORIENTED_EDGE ( 'NONE', *, *, #1594, .T. ) ;
#17421=FACE_OUTER_BOUND ( 'NONE', #15271, .T. ) ;
#17423=VECTOR ( 'NONE', #8650, 1000.000000000000000 ) ;
#17428=CARTESIAN_POINT ( 'NONE',  ( 0.000000000000000000, 0.000000000000000000, 0.000000000000000000 ) ) ;
#17433=DIRECTION ( 'NONE',  ( 0.000000000000000000, 0.000000000000000000, 1.000000000000000000 ) ) ;
#17436=DIRECTION ( 'NONE',  ( 1.000000000000000000, 0.000000000000000000, 0.000000000000000000 ) ) ;
#17437=DIRECTION ( 'NONE',  ( 0.000000000000000000, 0.000000000000000000, 1.000000000000000000 ) ) ;
#17452=CYLINDRICAL_SURFACE ( 'NONE', #15223, 1.000000000000002665 ) ;
#17454=AXIS2_PLACEMENT_3D ( 'NONE', #17216, #9728, #3703 ) ;
#17457=EDGE_LOOP ( 'NONE', ( #10466, #7617, #1783, #18005 ) ) ;
#17461=ORIENTED_EDGE ( 'NONE', *, *, #19221, .F. ) ;
#17467=AXIS2_PLACEMENT_3D ( 'NONE', #341, #6420, #12557 ) ;
#17469=ORIENTED_EDGE ( 'NONE', *, *, #5198, .T. ) ;
#17474=VECTOR ( 'NONE', #11396, 1000.000000000000000 ) ;
#17478=AXIS2_PLACEMENT_3D ( 'NONE', #18927, #8324, #17436 ) ;
#17479=ORIENTED_EDGE ( 'NONE', *, *, #15178, .F. ) ;
#17484=CARTESIAN_POINT ( 'NONE',  ( 2.255998204157473097, -17.85806462366060288, -32.00000000000000000 ) ) ;
#17485=VERTEX_POINT ( 'NONE', #4489 ) ;
#17488=EDGE_LOOP ( 'NONE', ( #7385, #18822 ) ) ;
#17492=PLANE ( 'NONE',  #8700 ) ;
#17496=CARTESIAN_POINT ( 'NONE',  ( -13.86923836996420967, -11.47363181547641275, -32.00000000000000000 ) ) ;
#17499=ORIENTED_EDGE ( 'NONE', *, *, #8757, .F. ) ;
#17505=AXIS2_PLACEMENT_3D ( 'NONE', #2414, #10132, #3921 ) ;
#17506=LINE ( 'NONE', #10013, #9246 ) ;
#17518=DIRECTION ( 'NONE',  ( 0.000000000000000000, 0.000000000000000000, -1.000000000000000000 ) ) ;
#17520=VERTEX_POINT ( 'NONE', #3088 ) ;
#17528=VERTEX_POINT ( 'NONE', #1401 ) ;
#17531=CARTESIAN_POINT ( 'NONE',  ( 16.68117051311640253, -3.372863662543048591, 35.00000000000000000 ) ) ;
#17535=CIRCLE ( 'NONE', #3784, 1.000000000000002665 ) ;
#17542=EDGE_CURVE ( 'NONE', #18804, #17931, #5981, .T. ) ;
#17543=DIRECTION ( 'NONE',  ( -1.000000000000000000, 0.000000000000000000, 0.000000000000000000 ) ) ;
#17544=DIRECTION ( 'NONE',  ( 1.000000000000000000, 0.000000000000000000, 0.000000000000000000 ) ) ;
#17563=EDGE_LOOP ( 'NONE', ( #17694, #3677 ) ) ;
#17569=DIRECTION ( 'NONE',  ( -0.000000000000000000, -0.000000000000000000, 1.000000000000000000 ) ) ;
#17570=EDGE_CURVE ( 'NONE', #12690, #13049, #2262, .T. ) ;
#17571=CARTESIAN_POINT ( 'NONE',  ( 14.19790265903627180, 9.644882309621939598, 35.00000000000000000 ) ) ;
#17583=CARTESIAN_POINT ( 'NONE',  ( -16.96448111170888851, 1.130229351527647585, 32.00000000000000000 ) ) ;
#17585=ORIENTED_EDGE ( 'NONE', *, *, #13211, .T. ) ;
#17588=ADVANCED_FACE ( 'NONE', ( #11091 ), #18686, .F. ) ;
#17593=CARTESIAN_POINT ( 'NONE',  ( 22.00000000000000355, 0.000000000000000000, 32.00000000000000000 ) ) ;
#17602=DIRECTION ( 'NONE',  ( -1.000000000000000000, 0.000000000000000000, 0.000000000000000000 ) ) ;
#17605=ORIENTED_EDGE ( 'NONE', *, *, #18735, .F. ) ;
#17606=CYLINDRICAL_SURFACE ( 'NONE', #15394, 0.9999999999999974465 ) ;
#17607=EDGE_CURVE ( 'NONE', #1381, #3988, #383, .T. ) ;
#17611=DIRECTION ( 'NONE',  ( -1.000000000000000000, 0.000000000000000000, 0.000000000000000000 ) ) ;
#17619=CARTESIAN_POINT ( 'NONE',  ( 14.86923836996420434, -11.47363181547641453, 32.00000000000000000 ) ) ;
#17622=AXIS2_PLACEMENT_3D ( 'NONE', #8435, #14333, #11525 ) ;
#17623=ORIENTED_EDGE ( 'NONE', *, *, #12734, .T. ) ;
#17630=CARTESIAN_POINT ( 'NONE',  ( -17.68117051311639898, -3.372863662543042818, 35.00000000000000000 ) ) ;
#17632=DIRECTION ( 'NONE',  ( 0.000000000000000000, 0.000000000000000000, 1.000000000000000000 ) ) ;
#17633=LINE ( 'NONE', #16035, #16830 ) ;
#17636=CIRCLE ( 'NONE', #5787, 1.000000000000004441 ) ;
#17639=DIRECTION ( 'NONE',  ( 1.000000000000000000, 0.000000000000000000, 0.000000000000000000 ) ) ;
#17640=DIRECTION ( 'NONE',  ( 0.000000000000000000, 0.000000000000000000, 1.000000000000000000 ) ) ;
#17645=FACE_BOUND ( 'NONE', #2267, .T. ) ;
#17647=DIRECTION ( 'NONE',  ( -0.000000000000000000, -0.000000000000000000, 1.000000000000000000 ) ) ;
#17649=ORIENTED_EDGE ( 'NONE', *, *, #18728, .T. ) ;
#17653=CARTESIAN_POINT ( 'NONE',  ( -5.476417968967388639, 17.43449690031536292, -32.00000000000000000 ) ) ;
#17668=DIRECTION ( 'NONE',  ( 1.000000000000000000, 0.000000000000000000, 0.000000000000000000 ) ) ;
#17673=CARTESIAN_POINT ( 'NONE',  ( 17.96448111170888851, 1.130229351527639148, 32.00000000000000000 ) ) ;
#17674=ADVANCED_FACE ( 'NONE', ( #9501 ), #14393, .T. ) ;
#17676=EDGE_LOOP ( 'NONE', ( #857, #7659, #10705, #996 ) ) ;
#17680=DIRECTION ( 'NONE',  ( 0.000000000000000000, 0.000000000000000000, 1.000000000000000000 ) ) ;
#17684=CARTESIAN_POINT ( 'NONE',  ( -9.580134541264520465, -14.56230589874905235, 32.00000000000000000 ) ) ;
#17693=AXIS2_PLACEMENT_3D ( 'NONE', #15694, #4696, #6465 ) ;
#17694=ORIENTED_EDGE ( 'NONE', *, *, #13356, .T. ) ;
#17695=DIRECTION ( 'NONE',  ( 0.000000000000000000, 0.000000000000000000, 1.000000000000000000 ) ) ;
#17704=DIRECTION ( 'NONE',  ( -1.000000000000000000, 0.000000000000000000, 0.000000000000000000 ) ) ;
#17716=DIRECTION ( 'NONE',  ( 0.000000000000000000, 0.000000000000000000, 1.000000000000000000 ) ) ;
#17719=ORIENTED_EDGE ( 'NONE', *, *, #13778, .T. ) ;
#17721=EDGE_LOOP ( 'NONE', ( #5704, #12567 ) ) ;
#17730=FACE_BOUND ( 'NONE', #2837, .T. ) ;
#17743=CARTESIAN_POINT ( 'NONE',  ( -16.96448111170888851, 1.130229351527647585, 35.00000000000000000 ) ) ;
#17745=ORIENTED_EDGE ( 'NONE', *, *, #3164, .F. ) ;
#17749=ORIENTED_EDGE ( 'NONE', *, *, #2669, .T. ) ;
#17750=CARTESIAN_POINT ( 'NONE',  ( -4.476417968967385974, 17.43449690031536292, -32.00000000000000000 ) ) ;
#17751=CARTESIAN_POINT ( 'NONE',  ( 9.000000000000000000, 0.000000000000000000, 29.00000000000000355 ) ) ;
#17752=EDGE_CURVE ( 'NONE', #5897, #4232, #4832, .T. ) ;
#17754=VERTEX_POINT ( 'NONE', #19447 ) ;
#17755=EDGE_CURVE ( 'NONE', #9521, #3237, #18263, .T. ) ;
#17757=CIRCLE ( 'NONE', #2735, 0.9999999999999974465 ) ;
#17759=AXIS2_PLACEMENT_3D ( 'NONE', #12984, #15982, #3867 ) ;
#17772=CIRCLE ( 'NONE', #10747, 1.000000000000000000 ) ;
#17774=CIRCLE ( 'NONE', #8185, 9.000000000000001776 ) ;
#17775=ORIENTED_EDGE ( 'NONE', *, *, #1956, .T. ) ;
#17779=CARTESIAN_POINT ( 'NONE',  ( -12.32184790671639085, 13.12143529358541549, -32.00000000000000000 ) ) ;
#17782=CARTESIAN_POINT ( 'NONE',  ( 16.68117051311640253, -3.372863662543048591, -32.00000000000000000 ) ) ;
#17783=ADVANCED_FACE ( 'NONE', ( #3679 ), #11754, .F. ) ;
#17784=CIRCLE ( 'NONE', #18101, 1.000000000000002665 ) ;
#17796=LINE ( 'NONE', #10496, #7029 ) ;
#17814=DIRECTION ( 'NONE',  ( 0.000000000000000000, 0.000000000000000000, 1.000000000000000000 ) ) ;
#17820=ORIENTED_EDGE ( 'NONE', *, *, #14344, .F. ) ;
#17824=EDGE_CURVE ( 'NONE', #271, #19757, #19543, .T. ) ;
#17830=VERTEX_POINT ( 'NONE', #9350 ) ;
#17835=DIRECTION ( 'NONE',  ( 0.000000000000000000, 0.000000000000000000, 1.000000000000000000 ) ) ;
#17836=FACE_BOUND ( 'NONE', #6925, .T. ) ;
#17850=ORIENTED_EDGE ( 'NONE', *, *, #19741, .F. ) ;
#17852=EDGE_CURVE ( 'NONE', #17485, #6807, #15051, .T. ) ;
#17855=VERTEX_POINT ( 'NONE', #38 ) ;
#17856=CARTESIAN_POINT ( 'NONE',  ( 17.11901729331276556, 5.562305898749055011, 32.00000000000000000 ) ) ;
#17859=DIRECTION ( 'NONE',  ( 0.000000000000000000, 0.000000000000000000, 1.000000000000000000 ) ) ;
#17863=ORIENTED_EDGE ( 'NONE', *, *, #5198, .F. ) ;
#17892=DIRECTION ( 'NONE',  ( 0.000000000000000000, 0.000000000000000000, 1.000000000000000000 ) ) ;
#17899=CARTESIAN_POINT ( 'NONE',  ( 8.671566133830875600, 15.77352024078954784, 32.00000000000000000 ) ) ;
#17903=ORIENTED_EDGE ( 'NONE', *, *, #5543, .T. ) ;
#17904=LINE ( 'NONE', #7478, #3363 ) ;
#17905=EDGE_CURVE ( 'NONE', #18333, #14047, #3231, .T. ) ;
#17907=DIRECTION ( 'NONE',  ( 1.000000000000000000, 0.000000000000000000, 0.000000000000000000 ) ) ;
#17909=EDGE_LOOP ( 'NONE', ( #8090, #13961 ) ) ;
#17917=ORIENTED_EDGE ( 'NONE', *, *, #10476, .F. ) ;
#17931=VERTEX_POINT ( 'NONE', #6223 ) ;
#17940=FACE_BOUND ( 'NONE', #8262, .T. ) ;
#17942=CARTESIAN_POINT ( 'NONE',  ( -7.626241948324210540, -16.73597674598852336, -35.00000000000000000 ) ) ;
#17944=CARTESIAN_POINT ( 'NONE',  ( 2.255998204157473097, -17.85806462366060288, -35.00000000000000000 ) ) ;
#17945=ORIENTED_EDGE ( 'NONE', *, *, #9588, .F. ) ;
#17947=FACE_OUTER_BOUND ( 'NONE', #18395, .T. ) ;
#17950=VECTOR ( 'NONE', #19229, 1000.000000000000000 ) ;
#17953=ORIENTED_EDGE ( 'NONE', *, *, #11951, .F. ) ;
#17964=CARTESIAN_POINT ( 'NONE',  ( -8.671566133830875600, 15.77352024078954429, -32.00000000000000000 ) ) ;
#17966=DIRECTION ( 'NONE',  ( 1.000000000000000000, 0.000000000000000000, 0.000000000000000000 ) ) ;
#17972=CIRCLE ( 'NONE', #19228, 0.9999999999999974465 ) ;
#17974=EDGE_CURVE ( 'NONE', #8529, #5313, #7364, .T. ) ;
#17979=VECTOR ( 'NONE', #1176, 1000.000000000000000 ) ;
#17982=ORIENTED_EDGE ( 'NONE', *, *, #11282, .T. ) ;
#17985=AXIS2_PLACEMENT_3D ( 'NONE', #14410, #2098, #17602 ) ;
#17986=EDGE_LOOP ( 'NONE', ( #19452, #13921, #15085, #16765 ) ) ;
#17988=CARTESIAN_POINT ( 'NONE',  ( -6.626241948324210540, -16.73597674598852336, -35.00000000000000000 ) ) ;
#17994=DIRECTION ( 'NONE',  ( -1.000000000000000000, 0.000000000000000000, 0.000000000000000000 ) ) ;
#17999=FACE_BOUND ( 'NONE', #18762, .T. ) ;
#18005=ORIENTED_EDGE ( 'NONE', *, *, #17251, .F. ) ;
#18017=EDGE_CURVE ( 'NONE', #14278, #16953, #6733, .T. ) ;
#18031=DIRECTION ( 'NONE',  ( -1.000000000000000000, 0.000000000000000000, 0.000000000000000000 ) ) ;
#18039=AXIS2_PLACEMENT_3D ( 'NONE', #5260, #865, #2543 ) ;
#18041=ORIENTED_EDGE ( 'NONE', *, *, #6817, .F. ) ;
#18049=ORIENTED_EDGE ( 'NONE', *, *, #7786, .F. ) ;
#18050=DIRECTION ( 'NONE',  ( 0.000000000000000000, 0.000000000000000000, 1.000000000000000000 ) ) ;
#18056=ORIENTED_EDGE ( 'NONE', *, *, #9215, .F. ) ;
#18065=ORIENTED_EDGE ( 'NONE', *, *, #4518, .F. ) ;
#18072=CARTESIAN_POINT ( 'NONE',  ( 4.476417968967386862, 17.43449690031536292, -35.00000000000000000 ) ) ;
#18074=VERTEX_POINT ( 'NONE', #5232 ) ;
#18076=CARTESIAN_POINT ( 'NONE',  ( -14.86923836996421144, -11.47363181547641275, -35.00000000000000000 ) ) ;
#18081=ORIENTED_EDGE ( 'NONE', *, *, #16872, .F. ) ;
#18083=LINE ( 'NONE', #10580, #17979 ) ;
#18089=CYLINDRICAL_SURFACE ( 'NONE', #9671, 1.000000000000004441 ) ;
#18090=EDGE_CURVE ( 'NONE', #12547, #17754, #642, .T. ) ;
#18092=VERTEX_POINT ( 'NONE', #18740 ) ;
#18093=DIRECTION ( 'NONE',  ( 1.000000000000000000, 0.000000000000000000, 0.000000000000000000 ) ) ;
#18101=AXIS2_PLACEMENT_3D ( 'NONE', #12897, #12996, #3880 ) ;
#18103=FACE_OUTER_BOUND ( 'NONE', #16065, .T. ) ;
#18111=ORIENTED_EDGE ( 'NONE', *, *, #6150, .F. ) ;
#18115=ORIENTED_EDGE ( 'NONE', *, *, #1710, .F. ) ;
#18116=EDGE_CURVE ( 'NONE', #11695, #16740, #12506, .T. ) ;
#18122=DIRECTION ( 'NONE',  ( 0.000000000000000000, 0.000000000000000000, 1.000000000000000000 ) ) ;
#18123=DIRECTION ( 'NONE',  ( 0.000000000000000000, 0.000000000000000000, -1.000000000000000000 ) ) ;
#18127=ADVANCED_FACE ( 'NONE', ( #15947 ), #12946, .F. ) ;
#18130=CIRCLE ( 'NONE', #16865, 0.9999999999999974465 ) ;
#18131=EDGE_CURVE ( 'NONE', #12048, #344, #13150, .T. ) ;
#18146=FACE_OUTER_BOUND ( 'NONE', #16467, .T. ) ;
#18148=AXIS2_PLACEMENT_3D ( 'NONE', #2872, #8986, #11688 ) ;
#18153=DIRECTION ( 'NONE',  ( 0.000000000000000000, 0.000000000000000000, -1.000000000000000000 ) ) ;
#18158=EDGE_CURVE ( 'NONE', #9320, #18721, #9659, .T. ) ;
#18162=ORIENTED_EDGE ( 'NONE', *, *, #13955, .F. ) ;
#18163=CYLINDRICAL_SURFACE ( 'NONE', #350, 0.9999999999999974465 ) ;
#18167=ORIENTED_EDGE ( 'NONE', *, *, #14108, .T. ) ;
#18172=ORIENTED_EDGE ( 'NONE', *, *, #11494, .T. ) ;
#18178=CIRCLE ( 'NONE', #907, 1.000000000000002665 ) ;
#18180=ORIENTED_EDGE ( 'NONE', *, *, #13955, .T. ) ;
#18187=CARTESIAN_POINT ( 'NONE',  ( -1.255998204157475318, -17.85806462366060288, 32.00000000000000000 ) ) ;
#18188=CIRCLE ( 'NONE', #613, 1.000000000000000888 ) ;
#18190=EDGE_CURVE ( 'NONE', #15562, #11187, #5148, .T. ) ;
#18193=VERTEX_POINT ( 'NONE', #3930 ) ;
#18194=CYLINDRICAL_SURFACE ( 'NONE', #18148, 1.000000000000000888 ) ;
#18197=DIRECTION ( 'NONE',  ( 1.000000000000000000, 0.000000000000000000, 0.000000000000000000 ) ) ;
#18203=ORIENTED_EDGE ( 'NONE', *, *, #3337, .T. ) ;
#18205=EDGE_CURVE ( 'NONE', #8877, #10068, #16331, .T. ) ;
#18212=ORIENTED_EDGE ( 'NONE', *, *, #7522, .F. ) ;
#18214=CARTESIAN_POINT ( 'NONE',  ( 13.86923836996420789, -11.47363181547641453, -32.00000000000000000 ) ) ;
#18216=ORIENTED_EDGE ( 'NONE', *, *, #19424, .F. ) ;
#18217=CYLINDRICAL_SURFACE ( 'NONE', #12392, 0.9999999999999974465 ) ;
#18222=EDGE_CURVE ( 'NONE', #11827, #7344, #19532, .T. ) ;
#18225=AXIS2_PLACEMENT_3D ( 'NONE', #19412, #19507, #4407 ) ;
#18231=EDGE_CURVE ( 'NONE', #3344, #11304, #18897, .T. ) ;
#18235=VERTEX_POINT ( 'NONE', #2420 ) ;
#18239=CARTESIAN_POINT ( 'NONE',  ( 12.00000000000000178, 1.469576158976824144E-15, 35.00000000000000000 ) ) ;
#18243=DIRECTION ( 'NONE',  ( 0.000000000000000000, 0.000000000000000000, 1.000000000000000000 ) ) ;
#18254=CARTESIAN_POINT ( 'NONE',  ( -15.19790265903627180, 9.644882309621941374, -35.00000000000000000 ) ) ;
#18260=EDGE_LOOP ( 'NONE', ( #7606, #18172, #4454, #14157 ) ) ;
#18263=CIRCLE ( 'NONE', #14753, 1.000000000000000888 ) ;
#18271=EDGE_CURVE ( 'NONE', #3690, #2257, #8035, .T. ) ;
#18272=ORIENTED_EDGE ( 'NONE', *, *, #1855, .T. ) ;
#18275=FACE_OUTER_BOUND ( 'NONE', #11126, .T. ) ;
#18279=CIRCLE ( 'NONE', #2612, 1.000000000000000888 ) ;
#18284=CARTESIAN_POINT ( 'NONE',  ( 0.000000000000000000, 0.000000000000000000, 32.00000000000000000 ) ) ;
#18286=DIRECTION ( 'NONE',  ( 0.000000000000000000, 0.000000000000000000, 1.000000000000000000 ) ) ;
#18295=DIRECTION ( 'NONE',  ( -0.000000000000000000, -0.000000000000000000, -1.000000000000000000 ) ) ;
#18305=DIRECTION ( 'NONE',  ( 0.000000000000000000, 0.000000000000000000, 1.000000000000000000 ) ) ;
#18310=FACE_OUTER_BOUND ( 'NONE', #18954, .T. ) ;
#18311=DIRECTION ( 'NONE',  ( -0.000000000000000000, -0.000000000000000000, 1.000000000000000000 ) ) ;
#18312=EDGE_LOOP ( 'NONE', ( #14841, #14875, #2036, #8538 ) ) ;
#18313=DIRECTION ( 'NONE',  ( 1.000000000000000000, 0.000000000000000000, 0.000000000000000000 ) ) ;
#18324=CARTESIAN_POINT ( 'NONE',  ( 13.86923836996420789, -11.47363181547641453, 35.00000000000000000 ) ) ;
#18333=VERTEX_POINT ( 'NONE', #4321 ) ;
#18334=CYLINDRICAL_SURFACE ( 'NONE', #13413, 1.000000000000002665 ) ;
#18336=CARTESIAN_POINT ( 'NONE',  ( 13.32184790671640151, 13.12143529358541016, 35.00000000000000000 ) ) ;
#18341=DIRECTION ( 'NONE',  ( 1.000000000000000000, 0.000000000000000000, 0.000000000000000000 ) ) ;
#18349=ORIENTED_EDGE ( 'NONE', *, *, #13292, .F. ) ;
#18352=EDGE_CURVE ( 'NONE', #13049, #12690, #11559, .T. ) ;
#18355=CARTESIAN_POINT ( 'NONE',  ( -4.476417968967385974, 17.43449690031536292, 32.00000000000000000 ) ) ;
#18361=ORIENTED_EDGE ( 'NONE', *, *, #19424, .T. ) ;
#18383=ORIENTED_EDGE ( 'NONE', *, *, #18513, .F. ) ;
#18395=EDGE_LOOP ( 'NONE', ( #6354, #16134, #2100, #12289 ) ) ;
#18399=CIRCLE ( 'NONE', #1152, 0.9999999999999974465 ) ;
#18404=DIRECTION ( 'NONE',  ( 0.000000000000000000, 0.000000000000000000, 1.000000000000000000 ) ) ;
#18411=DIRECTION ( 'NONE',  ( 0.000000000000000000, 0.000000000000000000, 1.000000000000000000 ) ) ;
#18412=ORIENTED_EDGE ( 'NONE', *, *, #11282, .F. ) ;
#18416=AXIS2_PLACEMENT_3D ( 'NONE', #1074, #8279, #14498 ) ;
#18421=EDGE_CURVE ( 'NONE', #15138, #1129, #19223, .T. ) ;
#18425=VECTOR ( 'NONE', #11196, 1000.000000000000000 ) ;
#18426=CARTESIAN_POINT ( 'NONE',  ( 0.000000000000000000, 0.000000000000000000, 29.00000000000000355 ) ) ;
#18428=AXIS2_PLACEMENT_3D ( 'NONE', #1976, #14185, #6559 ) ;
#18431=ORIENTED_EDGE ( 'NONE', *, *, #11774, .F. ) ;
#18435=DIRECTION ( 'NONE',  ( 1.000000000000000000, 0.000000000000000000, 0.000000000000000000 ) ) ;
#18442=VECTOR ( 'NONE', #18286, 1000.000000000000000 ) ;
#18443=FACE_OUTER_BOUND ( 'NONE', #14195, .T. ) ;
#18449=CYLINDRICAL_SURFACE ( 'NONE', #13234, 1.000000000000004441 ) ;
#18466=FACE_OUTER_BOUND ( 'NONE', #13805, .T. ) ;
#18467=CIRCLE ( 'NONE', #4415, 1.000000000000002665 ) ;
#18469=AXIS2_PLACEMENT_3D ( 'NONE', #110, #7292, #13515 ) ;
#18479=ORIENTED_EDGE ( 'NONE', *, *, #18352, .T. ) ;
#18481=CIRCLE ( 'NONE', #288, 1.000000000000004441 ) ;
#18496=CARTESIAN_POINT ( 'NONE',  ( 15.19790265903627358, 9.644882309621939598, 35.00000000000000000 ) ) ;
#18497=VERTEX_POINT ( 'NONE', #521 ) ;
#18509=EDGE_LOOP ( 'NONE', ( #11058, #44 ) ) ;
#18513=EDGE_CURVE ( 'NONE', #1230, #4750, #7811, .T. ) ;
#18514=VERTEX_POINT ( 'NONE', #9429 ) ;
#18516=DIRECTION ( 'NONE',  ( 0.000000000000000000, 0.000000000000000000, -1.000000000000000000 ) ) ;
#18526=EDGE_CURVE ( 'NONE', #10900, #11655, #6495, .T. ) ;
#18529=ORIENTED_EDGE ( 'NONE', *, *, #16300, .T. ) ;
#18549=CARTESIAN_POINT ( 'NONE',  ( -17.28688694438836393, -7.664027248171298545, -32.00000000000000000 ) ) ;
#18553=LINE ( 'NONE', #5244, #13824 ) ;
#18554=CYLINDRICAL_SURFACE ( 'NONE', #3218, 9.000000000000001776 ) ;
#18555=ORIENTED_EDGE ( 'NONE', *, *, #9215, .T. ) ;
#18561=LINE ( 'NONE', #8966, #2466 ) ;
#18563=ORIENTED_EDGE ( 'NONE', *, *, #4692, .T. ) ;
#18564=CYLINDRICAL_SURFACE ( 'NONE', #6760, 0.9999999999999974465 ) ;
#18579=CARTESIAN_POINT ( 'NONE',  ( -6.626241948324210540, -16.73597674598852336, 35.00000000000000000 ) ) ;
#18581=CARTESIAN_POINT ( 'NONE',  ( 5.510910596163084625E-16, 18.00000000000000355, 35.00000000000000000 ) ) ;
#18590=DIRECTION ( 'NONE',  ( 0.000000000000000000, 0.000000000000000000, 1.000000000000000000 ) ) ;
#18592=EDGE_CURVE ( 'NONE', #11187, #15562, #12540, .T. ) ;
#18593=DIRECTION ( 'NONE',  ( 1.000000000000000000, 0.000000000000000000, 0.000000000000000000 ) ) ;
#18595=VECTOR ( 'NONE', #13722, 1000.000000000000000 ) ;
#18596=CIRCLE ( 'NONE', #2625, 0.9999999999999974465 ) ;
#18600=CARTESIAN_POINT ( 'NONE',  ( -17.96448111170888851, 1.130229351527647585, -35.00000000000000000 ) ) ;
#18605=CARTESIAN_POINT ( 'NONE',  ( 10.58013454126452046, -14.56230589874905412, 32.00000000000000000 ) ) ;
#18614=AXIS2_PLACEMENT_3D ( 'NONE', #12049, #18153, #16647 ) ;
#18620=DIRECTION ( 'NONE',  ( 0.000000000000000000, 0.000000000000000000, -1.000000000000000000 ) ) ;
#18621=EDGE_LOOP ( 'NONE', ( #1861, #16770, #151, #1848 ) ) ;
#18625=VERTEX_POINT ( 'NONE', #6891 ) ;
#18629=ORIENTED_EDGE ( 'NONE', *, *, #17974, .T. ) ;
#18632=FACE_OUTER_BOUND ( 'NONE', #8693, .T. ) ;
#18636=AXIS2_PLACEMENT_3D ( 'NONE', #6779, #2092, #8195 ) ;
#18640=VERTEX_POINT ( 'NONE', #7178 ) ;
#18642=DIRECTION ( 'NONE',  ( -0.000000000000000000, -0.000000000000000000, 1.000000000000000000 ) ) ;
#18644=VERTEX_POINT ( 'NONE', #13300 ) ;
#18652=DIRECTION ( 'NONE',  ( -0.000000000000000000, -0.000000000000000000, 1.000000000000000000 ) ) ;
#18666=EDGE_CURVE ( 'NONE', #13990, #562, #19236, .T. ) ;
#18670=ORIENTED_EDGE ( 'NONE', *, *, #18090, .F. ) ;
#18674=AXIS2_PLACEMENT_3D ( 'NONE', #19115, #17716, #7183 ) ;
#18679=CARTESIAN_POINT ( 'NONE',  ( 0.000000000000000000, 0.000000000000000000, 32.00000000000000000 ) ) ;
#18684=ORIENTED_EDGE ( 'NONE', *, *, #9100, .F. ) ;
#18686=CYLINDRICAL_SURFACE ( 'NONE', #16320, 1.000000000000002442 ) ;
#18687=EDGE_CURVE ( 'NONE', #14452, #18235, #4200, .T. ) ;
#18688=FACE_OUTER_BOUND ( 'NONE', #7241, .T. ) ;
#18689=DIRECTION ( 'NONE',  ( 1.000000000000000000, 0.000000000000000000, 0.000000000000000000 ) ) ;
#18694=DIRECTION ( 'NONE',  ( 1.000000000000000000, 0.000000000000000000, 0.000000000000000000 ) ) ;
#18698=CARTESIAN_POINT ( 'NONE',  ( 14.00000000000000178, 1.714505518806294835E-15, 32.00000000000000000 ) ) ;
#18700=CARTESIAN_POINT ( 'NONE',  ( 7.671566133830872047, 15.77352024078954784, -32.00000000000000000 ) ) ;
#18702=CARTESIAN_POINT ( 'NONE',  ( 12.32184790671639618, 13.12143529358541016, 32.00000000000000000 ) ) ;
#18709=AXIS2_PLACEMENT_3D ( 'NONE', #4436, #5631, #13254 ) ;
#18721=VERTEX_POINT ( 'NONE', #16411 ) ;
#18728=EDGE_CURVE ( 'NONE', #11304, #3344, #16053, .T. ) ;
#18730=CARTESIAN_POINT ( 'NONE',  ( 9.580134541264516912, -14.56230589874905412, -32.00000000000000000 ) ) ;
#18735=EDGE_CURVE ( 'NONE', #16271, #155, #10508, .T. ) ;
#18737=LINE ( 'NONE', #17241, #15444 ) ;
#18740=CARTESIAN_POINT ( 'NONE',  ( 14.86923836996420434, -11.47363181547641453, -32.00000000000000000 ) ) ;
#18742=EDGE_CURVE ( 'NONE', #7627, #6438, #15308, .T. ) ;
#18752=EDGE_CURVE ( 'NONE', #2248, #9739, #15208, .T. ) ;
#18762=EDGE_LOOP ( 'NONE', ( #1543, #16776 ) ) ;
#18766=DIRECTION ( 'NONE',  ( 0.000000000000000000, 0.000000000000000000, 1.000000000000000000 ) ) ;
#18772=EDGE_LOOP ( 'NONE', ( #12865, #11737, #7995, #4128 ) ) ;
#18788=EDGE_CURVE ( 'NONE', #2678, #2901, #15405, .T. ) ;
#18790=DIRECTION ( 'NONE',  ( -0.000000000000000000, -0.000000000000000000, 1.000000000000000000 ) ) ;
#18792=CIRCLE ( 'NONE', #19127, 1.000000000000004441 ) ;
#18804=VERTEX_POINT ( 'NONE', #8081 ) ;
#18815=CARTESIAN_POINT ( 'NONE',  ( 18.96448111170889206, 1.130229351527639370, -32.00000000000000000 ) ) ;
#18821=EDGE_CURVE ( 'NONE', #3249, #1207, #10623, .T. ) ;
#18822=ORIENTED_EDGE ( 'NONE', *, *, #4637, .F. ) ;
#18830=DIRECTION ( 'NONE',  ( -1.000000000000000000, 0.000000000000000000, 0.000000000000000000 ) ) ;
#18831=CARTESIAN_POINT ( 'NONE',  ( -2.255998204157477538, -17.85806462366060288, 32.00000000000000000 ) ) ;
#18834=ADVANCED_FACE ( 'NONE', ( #18688 ), #6370, .F. ) ;
#18841=DIRECTION ( 'NONE',  ( 1.000000000000000000, 0.000000000000000000, 0.000000000000000000 ) ) ;
#18844=AXIS2_PLACEMENT_3D ( 'NONE', #13311, #943, #1511 ) ;
#18849=LINE ( 'NONE', #1939, #14527 ) ;
#18855=ORIENTED_EDGE ( 'NONE', *, *, #15007, .F. ) ;
#18861=ADVANCED_FACE ( 'NONE', ( #7981 ), #10995, .F. ) ;
#18866=ADVANCED_FACE ( 'NONE', ( #18889 ), #17195, .T. ) ;
#18869=FACE_BOUND ( 'NONE', #16567, .T. ) ;
#18872=LINE ( 'NONE', #7211, #7231 ) ;
#18875=STYLED_ITEM ( 'NONE', ( #4993 ), #15876 ) ;
#18883=CARTESIAN_POINT ( 'NONE',  ( -13.86923836996420967, -11.47363181547641275, 32.00000000000000000 ) ) ;
#18886=ORIENTED_EDGE ( 'NONE', *, *, #124, .F. ) ;
#18889=FACE_OUTER_BOUND ( 'NONE', #1058, .T. ) ;
#18891=DIRECTION ( 'NONE',  ( -0.000000000000000000, -0.000000000000000000, 1.000000000000000000 ) ) ;
#18894=DIRECTION ( 'NONE',  ( 1.000000000000000000, 0.000000000000000000, 0.000000000000000000 ) ) ;
#18896=CARTESIAN_POINT ( 'NONE',  ( 22.00000000000000355, 2.694222958124177204E-15, -32.00000000000000000 ) ) ;
#18897=CIRCLE ( 'NONE', #14441, 1.000000000000002665 ) ;
#18907=CARTESIAN_POINT ( 'NONE',  ( -14.19790265903626647, 9.644882309621941374, -32.00000000000000000 ) ) ;
#18917=DIRECTION ( 'NONE',  ( 1.000000000000000000, 0.000000000000000000, 0.000000000000000000 ) ) ;
#18921=EDGE_LOOP ( 'NONE', ( #17863, #5369 ) ) ;
#18924=CARTESIAN_POINT ( 'NONE',  ( 17.68117051311639898, -3.372863662543048591, 35.00000000000000000 ) ) ;
#18927=CARTESIAN_POINT ( 'NONE',  ( 8.671566133830875600, 15.77352024078954784, 32.00000000000000000 ) ) ;
#18933=PLANE ( 'NONE',  #3874 ) ;
#18934=DIRECTION ( 'NONE',  ( 0.000000000000000000, 0.000000000000000000, 1.000000000000000000 ) ) ;
#18946=CARTESIAN_POINT ( 'NONE',  ( -17.11901729331276911, 5.562305898749051458, -32.00000000000000000 ) ) ;
#18948=ORIENTED_EDGE ( 'NONE', *, *, #8569, .T. ) ;
#18953=VECTOR ( 'NONE', #13249, 1000.000000000000000 ) ;
#18954=EDGE_LOOP ( 'NONE', ( #13592, #7511, #7101, #3547 ) ) ;
#18962=EDGE_CURVE ( 'NONE', #18640, #9108, #13818, .T. ) ;
#18963=ORIENTED_EDGE ( 'NONE', *, *, #18742, .T. ) ;
#18964=AXIS2_PLACEMENT_3D ( 'NONE', #12695, #10897, #9707 ) ;
#18965=ADVANCED_FACE ( 'NONE', ( #6963, #2377 ), #17492, .F. ) ;
#18976=LINE ( 'NONE', #2269, #5056 ) ;
#18984=AXIS2_PLACEMENT_3D ( 'NONE', #2845, #1355, #7434 ) ;
#18990=AXIS2_PLACEMENT_3D ( 'NONE', #10608, #16610, #4304 ) ;
#18994=LINE ( 'NONE', #8393, #18425 ) ;
#18996=DIRECTION ( 'NONE',  ( 0.000000000000000000, 0.000000000000000000, 1.000000000000000000 ) ) ;
#18999=CARTESIAN_POINT ( 'NONE',  ( -10.58013454126452224, -14.56230589874905235, 32.00000000000000000 ) ) ;
#19011=FACE_OUTER_BOUND ( 'NONE', #17676, .T. ) ;
#19015=CIRCLE ( 'NONE', #5271, 0.9999999999999974465 ) ;
#19018=ORIENTED_EDGE ( 'NONE', *, *, #17852, .F. ) ;
#19026=ORIENTED_EDGE ( 'NONE', *, *, #17974, .F. ) ;
#19033=AXIS2_PLACEMENT_3D ( 'NONE', #17484, #13078, #14386 ) ;
#19034=ORIENTED_EDGE ( 'NONE', *, *, #8634, .F. ) ;
#19035=FACE_BOUND ( 'NONE', #13246, .T. ) ;
#19039=DIRECTION ( 'NONE',  ( 0.000000000000000000, 0.000000000000000000, -1.000000000000000000 ) ) ;
#19043=CARTESIAN_POINT ( 'NONE',  ( -7.671566133830872047, 15.77352024078954429, -35.00000000000000000 ) ) ;
#19054=VERTEX_POINT ( 'NONE', #8676 ) ;
#19057=FACE_OUTER_BOUND ( 'NONE', #5801, .T. ) ;
#19059=ADVANCED_FACE ( 'NONE', ( #9904 ), #14785, .F. ) ;
#19060=AXIS2_PLACEMENT_3D ( 'NONE', #10308, #13103, #1098 ) ;
#19064=EDGE_LOOP ( 'NONE', ( #6533, #5751 ) ) ;
#19069=EDGE_LOOP ( 'NONE', ( #7823, #4635, #5848, #12216 ) ) ;
#19071=EDGE_CURVE ( 'NONE', #6388, #3148, #11586, .T. ) ;
#19075=CARTESIAN_POINT ( 'NONE',  ( -15.19790265903627180, 9.644882309621941374, 32.00000000000000000 ) ) ;
#19083=AXIS2_PLACEMENT_3D ( 'NONE', #9516, #9416, #15514 ) ;
#19087=LINE ( 'NONE', #17593, #17474 ) ;
#19090=ORIENTED_EDGE ( 'NONE', *, *, #6884, .F. ) ;
#19094=DIRECTION ( 'NONE',  ( 1.000000000000000000, 0.000000000000000000, 0.000000000000000000 ) ) ;
#19100=ORIENTED_EDGE ( 'NONE', *, *, #6817, .T. ) ;
#19101=EDGE_CURVE ( 'NONE', #7536, #18514, #14788, .T. ) ;
#19104=LINE ( 'NONE', #10109, #1495 ) ;
#19107=DIRECTION ( 'NONE',  ( 0.000000000000000000, 0.000000000000000000, 1.000000000000000000 ) ) ;
#19108=CARTESIAN_POINT ( 'NONE',  ( -3.476417968967383754, 17.43449690031536292, -35.00000000000000000 ) ) ;
#19115=CARTESIAN_POINT ( 'NONE',  ( -17.11901729331276911, 5.562305898749051458, 32.00000000000000000 ) ) ;
#19120=CARTESIAN_POINT ( 'NONE',  ( 13.86923836996420789, -11.47363181547641453, -35.00000000000000000 ) ) ;
#19127=AXIS2_PLACEMENT_3D ( 'NONE', #9266, #6241, #16969 ) ;
#19132=ORIENTED_EDGE ( 'NONE', *, *, #16529, .T. ) ;
#19135=DIRECTION ( 'NONE',  ( 0.000000000000000000, 0.000000000000000000, 1.000000000000000000 ) ) ;
#19136=CARTESIAN_POINT ( 'NONE',  ( -6.626241948324210540, -16.73597674598852336, 32.00000000000000000 ) ) ;
#19137=CIRCLE ( 'NONE', #10521, 1.000000000000002442 ) ;
#19142=EDGE_LOOP ( 'NONE', ( #12663, #1245 ) ) ;
#19143=DIRECTION ( 'NONE',  ( 0.000000000000000000, 0.000000000000000000, 1.000000000000000000 ) ) ;
#19145=ORIENTED_EDGE ( 'NONE', *, *, #127, .F. ) ;
#19148=FACE_OUTER_BOUND ( 'NONE', #2542, .T. ) ;
#19150=ORIENTED_EDGE ( 'NONE', *, *, #2662, .T. ) ;
#19155=CARTESIAN_POINT ( 'NONE',  ( 1.255998204157470211, -17.85806462366060288, 32.00000000000000000 ) ) ;
#19161=EDGE_LOOP ( 'NONE', ( #8683, #14972 ) ) ;
#19162=DIRECTION ( 'NONE',  ( -0.000000000000000000, -0.000000000000000000, 1.000000000000000000 ) ) ;
#19165=EDGE_CURVE ( 'NONE', #12820, #1041, #18083, .T. ) ;
#19174=DIRECTION ( 'NONE',  ( -1.000000000000000000, 0.000000000000000000, 0.000000000000000000 ) ) ;
#19176=VERTEX_POINT ( 'NONE', #3063 ) ;
#19177=CARTESIAN_POINT ( 'NONE',  ( -7.626241948324210540, -16.73597674598852336, -32.00000000000000000 ) ) ;
#19185=ORIENTED_EDGE ( 'NONE', *, *, #5000, .F. ) ;
#19195=EDGE_LOOP ( 'NONE', ( #13530, #1017 ) ) ;
#19200=LINE ( 'NONE', #8514, #16 ) ;
#19205=VECTOR ( 'NONE', #743, 1000.000000000000000 ) ;
#19209=VECTOR ( 'NONE', #7022, 1000.000000000000000 ) ;
#19215=CARTESIAN_POINT ( 'NONE',  ( 17.68117051311639898, -3.372863662543048591, 32.00000000000000000 ) ) ;
#19219=ORIENTED_EDGE ( 'NONE', *, *, #18271, .F. ) ;
#19220=FACE_BOUND ( 'NONE', #4444, .T. ) ;
#19221=EDGE_CURVE ( 'NONE', #19054, #15416, #2319, .T. ) ;
#19223=CIRCLE ( 'NONE', #16357, 1.000000000000002665 ) ;
#19226=VECTOR ( 'NONE', #4501, 1000.000000000000000 ) ;
#19227=ADVANCED_FACE ( 'NONE', ( #19674 ), #4275, .F. ) ;
#19228=AXIS2_PLACEMENT_3D ( 'NONE', #1084, #7160, #14508 ) ;
#19229=DIRECTION ( 'NONE',  ( 0.000000000000000000, 0.000000000000000000, 1.000000000000000000 ) ) ;
#19231=ORIENTED_EDGE ( 'NONE', *, *, #4434, .F. ) ;
#19235=DIRECTION ( 'NONE',  ( 0.000000000000000000, 0.000000000000000000, 1.000000000000000000 ) ) ;
#19236=CIRCLE ( 'NONE', #3585, 1.000000000000000888 ) ;
#19242=DIRECTION ( 'NONE',  ( 0.000000000000000000, 0.000000000000000000, -1.000000000000000000 ) ) ;
#19249=CIRCLE ( 'NONE', #2633, 1.000000000000002665 ) ;
#19251=AXIS2_PLACEMENT_3D ( 'NONE', #14503, #8285, #17397 ) ;
#19254=AXIS2_PLACEMENT_3D ( 'NONE', #12745, #8336, #5329 ) ;
#19263=DIRECTION ( 'NONE',  ( 1.000000000000000000, 0.000000000000000000, 0.000000000000000000 ) ) ;
#19273=EDGE_LOOP ( 'NONE', ( #8771, #2610 ) ) ;
#19291=ORIENTED_EDGE ( 'NONE', *, *, #19071, .T. ) ;
#19292=DIRECTION ( 'NONE',  ( 0.000000000000000000, 0.000000000000000000, 1.000000000000000000 ) ) ;
#19302=AXIS2_PLACEMENT_3D ( 'NONE', #13070, #14765, #2260 ) ;
#19311=CIRCLE ( 'NONE', #2376, 1.000000000000003553 ) ;
#19321=EDGE_LOOP ( 'NONE', ( #15244, #8847, #9864, #11772 ) ) ;
#19322=ADVANCED_FACE ( 'NONE', ( #4764 ), #15774, .F. ) ;
#19330=ORIENTED_EDGE ( 'NONE', *, *, #1955, .F. ) ;
#19345=ADVANCED_FACE ( 'NONE', ( #17077 ), #3367, .F. ) ;
#19347=CIRCLE ( 'NONE', #14248, 1.000000000000000000 ) ;
#19383=DIRECTION ( 'NONE',  ( 0.000000000000000000, 0.000000000000000000, 1.000000000000000000 ) ) ;
#19384=EDGE_CURVE ( 'NONE', #4160, #8623, #12674, .T. ) ;
#19387=ADVANCED_FACE ( 'NONE', ( #5060 ), #3558, .F. ) ;
#19400=CARTESIAN_POINT ( 'NONE',  ( -17.96448111170888851, 1.130229351527647585, -35.00000000000000000 ) ) ;
#19412=CARTESIAN_POINT ( 'NONE',  ( 10.58013454126452046, -14.56230589874905412, -32.00000000000000000 ) ) ;
#19417=EDGE_LOOP ( 'NONE', ( #10954, #8980, #625, #11575 ) ) ;
#19419=CARTESIAN_POINT ( 'NONE',  ( -13.86923836996420967, -11.47363181547641275, -32.00000000000000000 ) ) ;
#19420=DIRECTION ( 'NONE',  ( -1.000000000000000000, 0.000000000000000000, 0.000000000000000000 ) ) ;
#19421=VERTEX_POINT ( 'NONE', #1668 ) ;
#19422=CIRCLE ( 'NONE', #18469, 1.000000000000000888 ) ;
#19423=DIRECTION ( 'NONE',  ( 0.000000000000000000, 0.000000000000000000, 1.000000000000000000 ) ) ;
#19424=EDGE_CURVE ( 'NONE', #10056, #19582, #9273, .T. ) ;
#19427=EDGE_LOOP ( 'NONE', ( #19570, #8459 ) ) ;
#19430=VERTEX_POINT ( 'NONE', #9884 ) ;
#19432=ORIENTED_EDGE ( 'NONE', *, *, #11628, .F. ) ;
#19435=ORIENTED_EDGE ( 'NONE', *, *, #18352, .F. ) ;
#19447=CARTESIAN_POINT ( 'NONE',  ( -9.000000000000001776, 0.000000000000000000, -35.00000000000000000 ) ) ;
#19449=CARTESIAN_POINT ( 'NONE',  ( 5.510910596163084625E-16, 18.00000000000000355, 32.00000000000000000 ) ) ;
#19452=ORIENTED_EDGE ( 'NONE', *, *, #12322, .F. ) ;
#19454=CARTESIAN_POINT ( 'NONE',  ( 3.255998204157476206, -17.85806462366060288, 32.00000000000000000 ) ) ;
#19457=VERTEX_POINT ( 'NONE', #17571 ) ;
#19458=ORIENTED_EDGE ( 'NONE', *, *, #13187, .T. ) ;
#19462=EDGE_LOOP ( 'NONE', ( #15055, #1356 ) ) ;
#19477=CIRCLE ( 'NONE', #6061, 1.000000000000002665 ) ;
#19483=DIRECTION ( 'NONE',  ( 0.000000000000000000, 0.000000000000000000, -1.000000000000000000 ) ) ;
#19484=LINE ( 'NONE', #9092, #11828 ) ;
#19492=CARTESIAN_POINT ( 'NONE',  ( 17.96448111170888851, 1.130229351527639148, 32.00000000000000000 ) ) ;
#19493=AXIS2_PLACEMENT_3D ( 'NONE', #10513, #13506, #8909 ) ;
#19500=DIRECTION ( 'NONE',  ( 0.000000000000000000, 0.000000000000000000, -1.000000000000000000 ) ) ;
#19507=DIRECTION ( 'NONE',  ( 0.000000000000000000, 0.000000000000000000, -1.000000000000000000 ) ) ;
#19523=FACE_BOUND ( 'NONE', #13702, .T. ) ;
#19524=ORIENTED_EDGE ( 'NONE', *, *, #7337, .F. ) ;
#19532=CIRCLE ( 'NONE', #372, 1.000000000000004441 ) ;
#19537=DIRECTION ( 'NONE',  ( 1.000000000000000000, 0.000000000000000000, 0.000000000000000000 ) ) ;
#19543=LINE ( 'NONE', #6132, #12821 ) ;
#19546=AXIS2_PLACEMENT_3D ( 'NONE', #587, #6959, #9697 ) ;
#19548=CIRCLE ( 'NONE', #15741, 1.000000000000004441 ) ;
#19557=ORIENTED_EDGE ( 'NONE', *, *, #18158, .T. ) ;
#19570=ORIENTED_EDGE ( 'NONE', *, *, #2107, .T. ) ;
#19577=VECTOR ( 'NONE', #2208, 1000.000000000000000 ) ;
#19578=ORIENTED_EDGE ( 'NONE', *, *, #7683, .T. ) ;
#19582=VERTEX_POINT ( 'NONE', #9058 ) ;
#19585=DIRECTION ( 'NONE',  ( 0.000000000000000000, 0.000000000000000000, 1.000000000000000000 ) ) ;
#19589=CIRCLE ( 'NONE', #16731, 1.000000000000002665 ) ;
#19591=CARTESIAN_POINT ( 'NONE',  ( 0.000000000000000000, 0.000000000000000000, 35.00000000000000000 ) ) ;
#19595=CARTESIAN_POINT ( 'NONE',  ( 6.626241948324199882, -16.73597674598852691, -32.00000000000000000 ) ) ;
#19598=EDGE_LOOP ( 'NONE', ( #18167, #7780 ) ) ;
#19617=ADVANCED_FACE ( 'NONE', ( #10559 ), #4547, .F. ) ;
#19622=DIRECTION ( 'NONE',  ( -1.000000000000000000, 0.000000000000000000, 0.000000000000000000 ) ) ;
#19625=VECTOR ( 'NONE', #7230, 1000.000000000000000 ) ;
#19632=CIRCLE ( 'NONE', #18674, 1.000000000000000888 ) ;
#19638=ORIENTED_EDGE ( 'NONE', *, *, #1813, .F. ) ;
#19651=DIRECTION ( 'NONE',  ( 1.000000000000000000, 0.000000000000000000, 0.000000000000000000 ) ) ;
#19653=AXIS2_PLACEMENT_3D ( 'NONE', #17289, #14392, #8079 ) ;
#19654=FACE_OUTER_BOUND ( 'NONE', #7062, .T. ) ;
#19655=VECTOR ( 'NONE', #11447, 1000.000000000000000 ) ;
#19663=ORIENTED_EDGE ( 'NONE', *, *, #2231, .F. ) ;
#19674=FACE_OUTER_BOUND ( 'NONE', #8904, .T. ) ;
#19676=EDGE_CURVE ( 'NONE', #19176, #676, #14491, .T. ) ;
#19678=DIRECTION ( 'NONE',  ( 1.000000000000000000, 0.000000000000000000, 0.000000000000000000 ) ) ;
#19682=DIRECTION ( 'NONE',  ( -0.000000000000000000, -0.000000000000000000, 1.000000000000000000 ) ) ;
#19686=FACE_BOUND ( 'NONE', #5517, .T. ) ;
#19689=DIRECTION ( 'NONE',  ( 0.000000000000000000, 0.000000000000000000, 1.000000000000000000 ) ) ;
#19697=AXIS2_PLACEMENT_3D ( 'NONE', #11086, #5171, #6459 ) ;
#19704=DIRECTION ( 'NONE',  ( 0.000000000000000000, 0.000000000000000000, -1.000000000000000000 ) ) ;
#19705=VERTEX_POINT ( 'NONE', #1453 ) ;
#19707=CIRCLE ( 'NONE', #2776, 1.000000000000003553 ) ;
#19733=DIRECTION ( 'NONE',  ( -0.000000000000000000, -0.000000000000000000, 1.000000000000000000 ) ) ;
#19741=EDGE_CURVE ( 'NONE', #10790, #7654, #5014, .T. ) ;
#19756=EDGE_LOOP ( 'NONE', ( #8041, #8247 ) ) ;
#19757=VERTEX_POINT ( 'NONE', #8115 ) ;
#19777=DIRECTION ( 'NONE',  ( 0.000000000000000000, 0.000000000000000000, 1.000000000000000000 ) ) ;
#19779=CARTESIAN_POINT ( 'NONE',  ( -18.68117051311639543, -3.372863662543042818, -35.00000000000000000 ) ) ;
ENDSEC;
END-ISO-10303-21;
